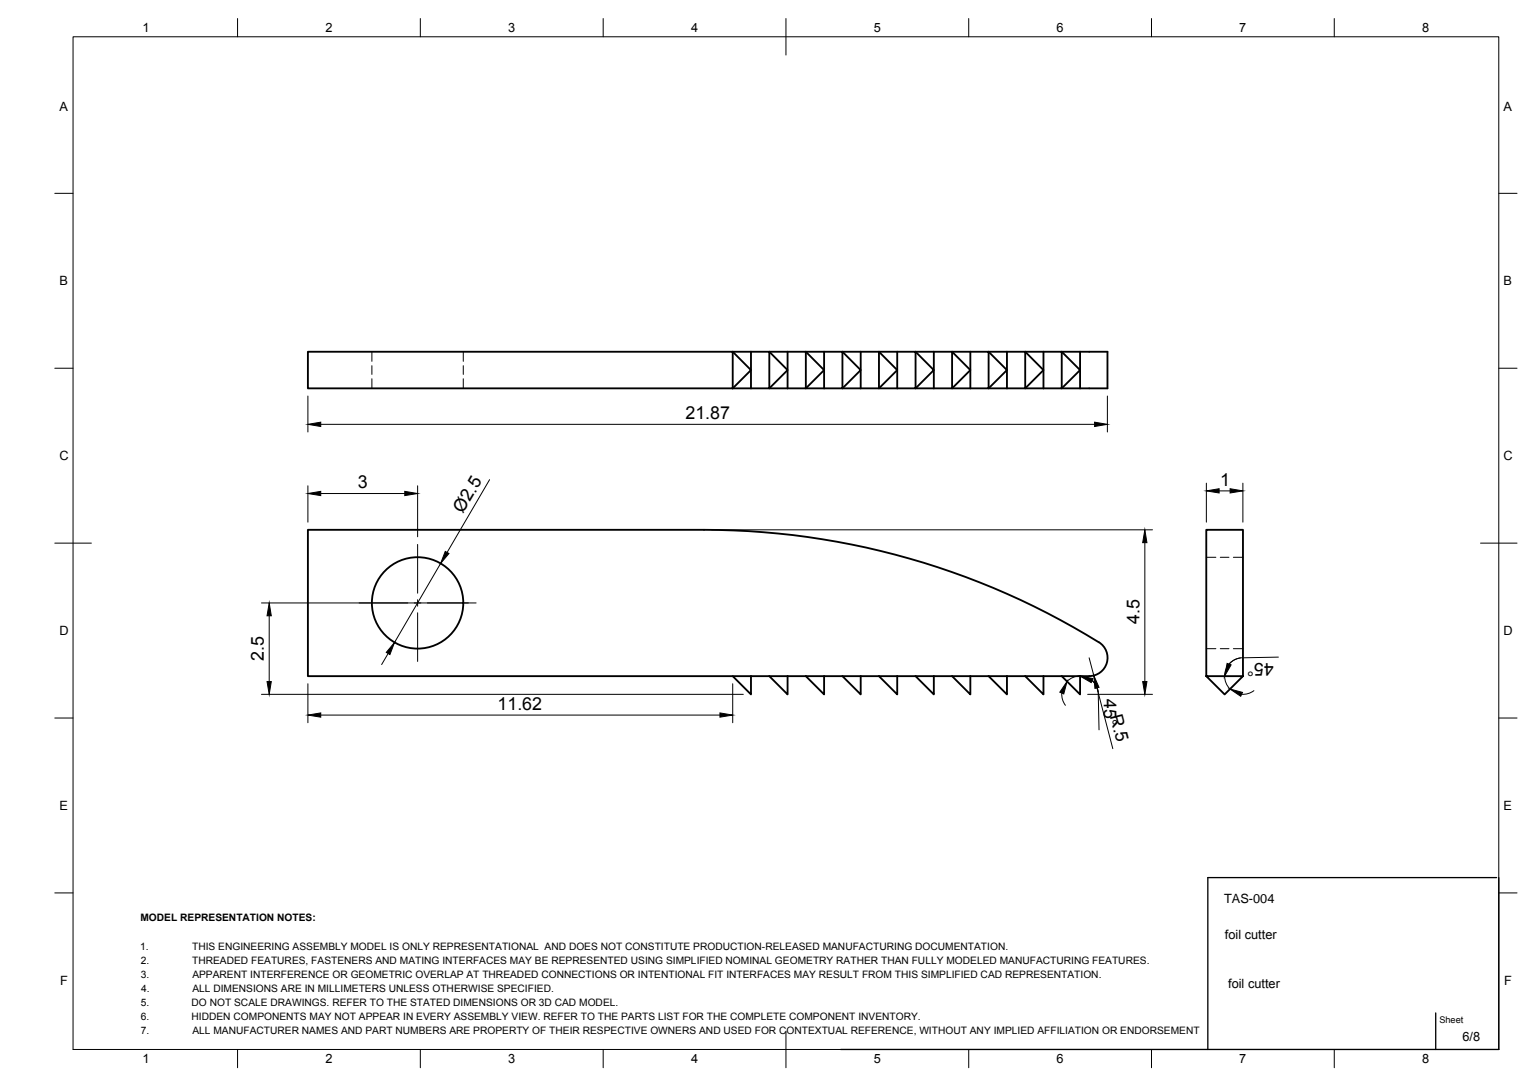
ISO-10303-21;
HEADER;
/* Generated by software containing ST-Developer
 * from STEP Tools, Inc. (www.steptools.com) 
 */

FILE_DESCRIPTION(
/* description */ ('STEP AP214'),
/* implementation_level */ '2;1');

FILE_NAME(
/* name */ 'foil cutter.step',
/* time_stamp */ '2026-11-04T19:48:07-08:00',
/* author */ (''),
/* organization */ (''),
/* preprocessor_version */ 'ST-DEVELOPER v20.2',
/* originating_system */ 'Autodesk Translation Framework v15.17.0.0',
/* authorisation */ '');

FILE_SCHEMA (('AUTOMOTIVE_DESIGN { 1 0 10303 214 3 1 1 }'));
ENDSEC;

DATA;
#10=MECHANICAL_DESIGN_GEOMETRIC_PRESENTATION_REPRESENTATION('',(#62),#9561);
#50=SHAPE_REPRESENTATION_RELATIONSHIP('SRR','None',#9590,#56);
#56=ADVANCED_BREP_SHAPE_REPRESENTATION('',(#68),#9558);
#62=STYLED_ITEM('',(#9626),#68);
#68=MANIFOLD_SOLID_BREP('Body1',#2408);
#84=FACE_BOUND('',#444,.T.);
#85=FACE_BOUND('',#446,.T.);
#135=PLANE('',#2617);
#136=PLANE('',#2618);
#137=PLANE('',#2619);
#138=PLANE('',#2620);
#139=PLANE('',#2621);
#140=PLANE('',#2622);
#141=PLANE('',#2623);
#142=PLANE('',#2624);
#143=PLANE('',#2625);
#144=PLANE('',#2626);
#145=PLANE('',#2627);
#146=PLANE('',#2628);
#147=PLANE('',#2629);
#148=PLANE('',#2630);
#149=PLANE('',#2633);
#150=PLANE('',#2638);
#151=PLANE('',#2639);
#152=PLANE('',#2640);
#153=PLANE('',#2641);
#154=PLANE('',#2642);
#155=PLANE('',#2643);
#156=PLANE('',#2644);
#157=PLANE('',#2645);
#158=PLANE('',#2646);
#159=PLANE('',#2647);
#160=PLANE('',#2648);
#161=PLANE('',#2649);
#162=PLANE('',#2650);
#163=PLANE('',#2651);
#164=PLANE('',#2652);
#165=PLANE('',#2653);
#166=PLANE('',#2654);
#167=PLANE('',#2655);
#168=PLANE('',#2656);
#169=PLANE('',#2657);
#170=PLANE('',#2658);
#171=PLANE('',#2659);
#172=PLANE('',#2660);
#173=PLANE('',#2661);
#174=PLANE('',#2662);
#175=PLANE('',#2663);
#176=PLANE('',#2664);
#177=PLANE('',#2665);
#178=PLANE('',#2666);
#179=PLANE('',#2667);
#180=PLANE('',#2668);
#181=PLANE('',#2669);
#182=PLANE('',#2670);
#183=PLANE('',#2671);
#184=PLANE('',#2672);
#185=PLANE('',#2673);
#186=PLANE('',#2674);
#187=PLANE('',#2675);
#188=PLANE('',#2676);
#189=PLANE('',#2677);
#273=FACE_OUTER_BOUND('',#429,.T.);
#274=FACE_OUTER_BOUND('',#430,.T.);
#275=FACE_OUTER_BOUND('',#431,.T.);
#276=FACE_OUTER_BOUND('',#432,.T.);
#277=FACE_OUTER_BOUND('',#433,.T.);
#278=FACE_OUTER_BOUND('',#434,.T.);
#279=FACE_OUTER_BOUND('',#435,.T.);
#280=FACE_OUTER_BOUND('',#436,.T.);
#281=FACE_OUTER_BOUND('',#437,.T.);
#282=FACE_OUTER_BOUND('',#438,.T.);
#283=FACE_OUTER_BOUND('',#439,.T.);
#284=FACE_OUTER_BOUND('',#440,.T.);
#285=FACE_OUTER_BOUND('',#441,.T.);
#286=FACE_OUTER_BOUND('',#442,.T.);
#287=FACE_OUTER_BOUND('',#443,.T.);
#288=FACE_OUTER_BOUND('',#445,.T.);
#289=FACE_OUTER_BOUND('',#447,.T.);
#290=FACE_OUTER_BOUND('',#448,.T.);
#291=FACE_OUTER_BOUND('',#449,.T.);
#292=FACE_OUTER_BOUND('',#450,.T.);
#293=FACE_OUTER_BOUND('',#451,.T.);
#294=FACE_OUTER_BOUND('',#452,.T.);
#295=FACE_OUTER_BOUND('',#453,.T.);
#296=FACE_OUTER_BOUND('',#454,.T.);
#297=FACE_OUTER_BOUND('',#455,.T.);
#298=FACE_OUTER_BOUND('',#456,.T.);
#299=FACE_OUTER_BOUND('',#457,.T.);
#300=FACE_OUTER_BOUND('',#458,.T.);
#301=FACE_OUTER_BOUND('',#459,.T.);
#302=FACE_OUTER_BOUND('',#460,.T.);
#303=FACE_OUTER_BOUND('',#461,.T.);
#304=FACE_OUTER_BOUND('',#462,.T.);
#305=FACE_OUTER_BOUND('',#463,.T.);
#306=FACE_OUTER_BOUND('',#464,.T.);
#307=FACE_OUTER_BOUND('',#465,.T.);
#308=FACE_OUTER_BOUND('',#466,.T.);
#309=FACE_OUTER_BOUND('',#467,.T.);
#310=FACE_OUTER_BOUND('',#468,.T.);
#311=FACE_OUTER_BOUND('',#469,.T.);
#312=FACE_OUTER_BOUND('',#470,.T.);
#313=FACE_OUTER_BOUND('',#471,.T.);
#314=FACE_OUTER_BOUND('',#472,.T.);
#315=FACE_OUTER_BOUND('',#473,.T.);
#316=FACE_OUTER_BOUND('',#474,.T.);
#317=FACE_OUTER_BOUND('',#475,.T.);
#318=FACE_OUTER_BOUND('',#476,.T.);
#319=FACE_OUTER_BOUND('',#477,.T.);
#320=FACE_OUTER_BOUND('',#478,.T.);
#321=FACE_OUTER_BOUND('',#479,.T.);
#322=FACE_OUTER_BOUND('',#480,.T.);
#323=FACE_OUTER_BOUND('',#481,.T.);
#324=FACE_OUTER_BOUND('',#482,.T.);
#325=FACE_OUTER_BOUND('',#483,.T.);
#326=FACE_OUTER_BOUND('',#484,.T.);
#327=FACE_OUTER_BOUND('',#485,.T.);
#328=FACE_OUTER_BOUND('',#486,.T.);
#329=FACE_OUTER_BOUND('',#487,.T.);
#330=FACE_OUTER_BOUND('',#488,.T.);
#429=EDGE_LOOP('',(#1983,#1984,#1985,#1986));
#430=EDGE_LOOP('',(#1987,#1988,#1989,#1990));
#431=EDGE_LOOP('',(#1991,#1992,#1993,#1994));
#432=EDGE_LOOP('',(#1995,#1996,#1997,#1998));
#433=EDGE_LOOP('',(#1999,#2000,#2001,#2002));
#434=EDGE_LOOP('',(#2003,#2004,#2005,#2006));
#435=EDGE_LOOP('',(#2007,#2008,#2009,#2010));
#436=EDGE_LOOP('',(#2011,#2012,#2013,#2014));
#437=EDGE_LOOP('',(#2015,#2016,#2017,#2018));
#438=EDGE_LOOP('',(#2019,#2020,#2021,#2022));
#439=EDGE_LOOP('',(#2023,#2024,#2025,#2026));
#440=EDGE_LOOP('',(#2027,#2028,#2029,#2030));
#441=EDGE_LOOP('',(#2031,#2032,#2033,#2034));
#442=EDGE_LOOP('',(#2035,#2036,#2037,#2038));
#443=EDGE_LOOP('',(#2039,#2040,#2041,#2042,#2043,#2044,#2045,#2046,#2047,
#2048,#2049,#2050,#2051,#2052,#2053,#2054,#2055,#2056,#2057,#2058,#2059,
#2060,#2061,#2062,#2063));
#444=EDGE_LOOP('',(#2064));
#445=EDGE_LOOP('',(#2065,#2066,#2067,#2068,#2069,#2070,#2071,#2072,#2073,
#2074,#2075,#2076,#2077,#2078,#2079,#2080,#2081,#2082,#2083,#2084,#2085,
#2086,#2087,#2088,#2089));
#446=EDGE_LOOP('',(#2090));
#447=EDGE_LOOP('',(#2091,#2092,#2093,#2094));
#448=EDGE_LOOP('',(#2095,#2096,#2097,#2098));
#449=EDGE_LOOP('',(#2099,#2100,#2101));
#450=EDGE_LOOP('',(#2102,#2103,#2104));
#451=EDGE_LOOP('',(#2105,#2106,#2107));
#452=EDGE_LOOP('',(#2108,#2109,#2110));
#453=EDGE_LOOP('',(#2111,#2112,#2113));
#454=EDGE_LOOP('',(#2114,#2115,#2116));
#455=EDGE_LOOP('',(#2117,#2118,#2119));
#456=EDGE_LOOP('',(#2120,#2121,#2122));
#457=EDGE_LOOP('',(#2123,#2124,#2125));
#458=EDGE_LOOP('',(#2126,#2127,#2128));
#459=EDGE_LOOP('',(#2129,#2130,#2131));
#460=EDGE_LOOP('',(#2132,#2133,#2134));
#461=EDGE_LOOP('',(#2135,#2136,#2137));
#462=EDGE_LOOP('',(#2138,#2139,#2140));
#463=EDGE_LOOP('',(#2141,#2142,#2143));
#464=EDGE_LOOP('',(#2144,#2145,#2146));
#465=EDGE_LOOP('',(#2147,#2148,#2149));
#466=EDGE_LOOP('',(#2150,#2151,#2152));
#467=EDGE_LOOP('',(#2153,#2154,#2155));
#468=EDGE_LOOP('',(#2156,#2157,#2158));
#469=EDGE_LOOP('',(#2159,#2160,#2161));
#470=EDGE_LOOP('',(#2162,#2163,#2164));
#471=EDGE_LOOP('',(#2165,#2166,#2167));
#472=EDGE_LOOP('',(#2168,#2169,#2170));
#473=EDGE_LOOP('',(#2171,#2172,#2173));
#474=EDGE_LOOP('',(#2174,#2175,#2176));
#475=EDGE_LOOP('',(#2177,#2178,#2179));
#476=EDGE_LOOP('',(#2180,#2181,#2182));
#477=EDGE_LOOP('',(#2183,#2184,#2185));
#478=EDGE_LOOP('',(#2186,#2187,#2188));
#479=EDGE_LOOP('',(#2189,#2190,#2191));
#480=EDGE_LOOP('',(#2192,#2193,#2194));
#481=EDGE_LOOP('',(#2195,#2196,#2197));
#482=EDGE_LOOP('',(#2198,#2199,#2200));
#483=EDGE_LOOP('',(#2201,#2202,#2203));
#484=EDGE_LOOP('',(#2204,#2205,#2206));
#485=EDGE_LOOP('',(#2207,#2208,#2209));
#486=EDGE_LOOP('',(#2210,#2211,#2212));
#487=EDGE_LOOP('',(#2213,#2214,#2215));
#488=EDGE_LOOP('',(#2216,#2217,#2218));
#631=LINE('',#9288,#881);
#632=LINE('',#9293,#882);
#633=LINE('',#9295,#883);
#634=LINE('',#9297,#884);
#635=LINE('',#9298,#885);
#636=LINE('',#9302,#886);
#637=LINE('',#9304,#887);
#638=LINE('',#9306,#888);
#639=LINE('',#9307,#889);
#640=LINE('',#9311,#890);
#641=LINE('',#9313,#891);
#642=LINE('',#9315,#892);
#643=LINE('',#9316,#893);
#644=LINE('',#9320,#894);
#645=LINE('',#9322,#895);
#646=LINE('',#9324,#896);
#647=LINE('',#9325,#897);
#648=LINE('',#9329,#898);
#649=LINE('',#9331,#899);
#650=LINE('',#9333,#900);
#651=LINE('',#9334,#901);
#652=LINE('',#9338,#902);
#653=LINE('',#9340,#903);
#654=LINE('',#9342,#904);
#655=LINE('',#9343,#905);
#656=LINE('',#9347,#906);
#657=LINE('',#9349,#907);
#658=LINE('',#9351,#908);
#659=LINE('',#9352,#909);
#660=LINE('',#9356,#910);
#661=LINE('',#9358,#911);
#662=LINE('',#9360,#912);
#663=LINE('',#9361,#913);
#664=LINE('',#9365,#914);
#665=LINE('',#9367,#915);
#666=LINE('',#9369,#916);
#667=LINE('',#9370,#917);
#668=LINE('',#9374,#918);
#669=LINE('',#9376,#919);
#670=LINE('',#9378,#920);
#671=LINE('',#9379,#921);
#672=LINE('',#9383,#922);
#673=LINE('',#9385,#923);
#674=LINE('',#9387,#924);
#675=LINE('',#9388,#925);
#676=LINE('',#9391,#926);
#677=LINE('',#9393,#927);
#678=LINE('',#9394,#928);
#679=LINE('',#9397,#929);
#680=LINE('',#9399,#930);
#681=LINE('',#9400,#931);
#682=LINE('',#9402,#932);
#683=LINE('',#9403,#933);
#684=LINE('',#9404,#934);
#685=LINE('',#9405,#935);
#686=LINE('',#9406,#936);
#687=LINE('',#9407,#937);
#688=LINE('',#9408,#938);
#689=LINE('',#9409,#939);
#690=LINE('',#9410,#940);
#691=LINE('',#9411,#941);
#692=LINE('',#9416,#942);
#693=LINE('',#9417,#943);
#694=LINE('',#9418,#944);
#695=LINE('',#9419,#945);
#696=LINE('',#9420,#946);
#697=LINE('',#9421,#947);
#698=LINE('',#9422,#948);
#699=LINE('',#9423,#949);
#700=LINE('',#9424,#950);
#701=LINE('',#9425,#951);
#702=LINE('',#9430,#952);
#703=LINE('',#9434,#953);
#704=LINE('',#9435,#954);
#705=LINE('',#9437,#955);
#706=LINE('',#9439,#956);
#707=LINE('',#9443,#957);
#708=LINE('',#9444,#958);
#709=LINE('',#9446,#959);
#710=LINE('',#9448,#960);
#711=LINE('',#9452,#961);
#712=LINE('',#9453,#962);
#713=LINE('',#9455,#963);
#714=LINE('',#9457,#964);
#715=LINE('',#9461,#965);
#716=LINE('',#9462,#966);
#717=LINE('',#9464,#967);
#718=LINE('',#9466,#968);
#719=LINE('',#9470,#969);
#720=LINE('',#9471,#970);
#721=LINE('',#9473,#971);
#722=LINE('',#9475,#972);
#723=LINE('',#9479,#973);
#724=LINE('',#9480,#974);
#725=LINE('',#9482,#975);
#726=LINE('',#9484,#976);
#727=LINE('',#9488,#977);
#728=LINE('',#9489,#978);
#729=LINE('',#9491,#979);
#730=LINE('',#9493,#980);
#731=LINE('',#9497,#981);
#732=LINE('',#9498,#982);
#733=LINE('',#9500,#983);
#734=LINE('',#9502,#984);
#735=LINE('',#9506,#985);
#736=LINE('',#9507,#986);
#737=LINE('',#9509,#987);
#738=LINE('',#9511,#988);
#739=LINE('',#9515,#989);
#740=LINE('',#9516,#990);
#741=LINE('',#9518,#991);
#742=LINE('',#9520,#992);
#881=VECTOR('',#3108,1.25);
#882=VECTOR('',#3113,1000.);
#883=VECTOR('',#3114,1000.);
#884=VECTOR('',#3115,1000.);
#885=VECTOR('',#3116,1000.);
#886=VECTOR('',#3119,1000.);
#887=VECTOR('',#3120,1000.);
#888=VECTOR('',#3121,1000.);
#889=VECTOR('',#3122,1000.);
#890=VECTOR('',#3125,1000.);
#891=VECTOR('',#3126,1000.);
#892=VECTOR('',#3127,1000.);
#893=VECTOR('',#3128,1000.);
#894=VECTOR('',#3131,1000.);
#895=VECTOR('',#3132,1000.);
#896=VECTOR('',#3133,1000.);
#897=VECTOR('',#3134,1000.);
#898=VECTOR('',#3137,1000.);
#899=VECTOR('',#3138,1000.);
#900=VECTOR('',#3139,1000.);
#901=VECTOR('',#3140,1000.);
#902=VECTOR('',#3143,1000.);
#903=VECTOR('',#3144,1000.);
#904=VECTOR('',#3145,1000.);
#905=VECTOR('',#3146,1000.);
#906=VECTOR('',#3149,1000.);
#907=VECTOR('',#3150,1000.);
#908=VECTOR('',#3151,1000.);
#909=VECTOR('',#3152,1000.);
#910=VECTOR('',#3155,1000.);
#911=VECTOR('',#3156,1000.);
#912=VECTOR('',#3157,1000.);
#913=VECTOR('',#3158,1000.);
#914=VECTOR('',#3161,1000.);
#915=VECTOR('',#3162,1000.);
#916=VECTOR('',#3163,1000.);
#917=VECTOR('',#3164,1000.);
#918=VECTOR('',#3167,1000.);
#919=VECTOR('',#3168,1000.);
#920=VECTOR('',#3169,1000.);
#921=VECTOR('',#3170,1000.);
#922=VECTOR('',#3173,1000.);
#923=VECTOR('',#3174,1000.);
#924=VECTOR('',#3175,1000.);
#925=VECTOR('',#3176,1000.);
#926=VECTOR('',#3179,1000.);
#927=VECTOR('',#3180,1000.);
#928=VECTOR('',#3181,1000.);
#929=VECTOR('',#3184,1000.);
#930=VECTOR('',#3185,1000.);
#931=VECTOR('',#3186,1000.);
#932=VECTOR('',#3189,1000.);
#933=VECTOR('',#3190,1000.);
#934=VECTOR('',#3191,1000.);
#935=VECTOR('',#3192,1000.);
#936=VECTOR('',#3193,1000.);
#937=VECTOR('',#3194,1000.);
#938=VECTOR('',#3195,1000.);
#939=VECTOR('',#3196,1000.);
#940=VECTOR('',#3197,1000.);
#941=VECTOR('',#3198,1000.);
#942=VECTOR('',#3205,1000.);
#943=VECTOR('',#3206,1000.);
#944=VECTOR('',#3207,1000.);
#945=VECTOR('',#3208,1000.);
#946=VECTOR('',#3209,1000.);
#947=VECTOR('',#3210,1000.);
#948=VECTOR('',#3211,1000.);
#949=VECTOR('',#3212,1000.);
#950=VECTOR('',#3213,1000.);
#951=VECTOR('',#3214,1000.);
#952=VECTOR('',#3221,1000.);
#953=VECTOR('',#3226,1000.);
#954=VECTOR('',#3227,1000.);
#955=VECTOR('',#3230,1000.);
#956=VECTOR('',#3233,1000.);
#957=VECTOR('',#3238,1000.);
#958=VECTOR('',#3239,1000.);
#959=VECTOR('',#3242,1000.);
#960=VECTOR('',#3245,1000.);
#961=VECTOR('',#3250,1000.);
#962=VECTOR('',#3251,1000.);
#963=VECTOR('',#3254,1000.);
#964=VECTOR('',#3257,1000.);
#965=VECTOR('',#3262,1000.);
#966=VECTOR('',#3263,1000.);
#967=VECTOR('',#3266,1000.);
#968=VECTOR('',#3269,1000.);
#969=VECTOR('',#3274,1000.);
#970=VECTOR('',#3275,1000.);
#971=VECTOR('',#3278,1000.);
#972=VECTOR('',#3281,1000.);
#973=VECTOR('',#3286,1000.);
#974=VECTOR('',#3287,1000.);
#975=VECTOR('',#3290,1000.);
#976=VECTOR('',#3293,1000.);
#977=VECTOR('',#3298,1000.);
#978=VECTOR('',#3299,1000.);
#979=VECTOR('',#3302,1000.);
#980=VECTOR('',#3305,1000.);
#981=VECTOR('',#3310,1000.);
#982=VECTOR('',#3311,1000.);
#983=VECTOR('',#3314,1000.);
#984=VECTOR('',#3317,1000.);
#985=VECTOR('',#3322,1000.);
#986=VECTOR('',#3323,1000.);
#987=VECTOR('',#3326,1000.);
#988=VECTOR('',#3329,1000.);
#989=VECTOR('',#3334,1000.);
#990=VECTOR('',#3335,1000.);
#991=VECTOR('',#3338,1000.);
#992=VECTOR('',#3341,1000.);
#1051=CIRCLE('',#2615,1.25);
#1052=CIRCLE('',#2616,1.25);
#1053=CIRCLE('',#2631,20.5);
#1054=CIRCLE('',#2632,0.5);
#1055=CIRCLE('',#2634,0.5);
#1056=CIRCLE('',#2635,20.5);
#1193=VERTEX_POINT('',#9285);
#1194=VERTEX_POINT('',#9287);
#1195=VERTEX_POINT('',#9291);
#1196=VERTEX_POINT('',#9292);
#1197=VERTEX_POINT('',#9294);
#1198=VERTEX_POINT('',#9296);
#1199=VERTEX_POINT('',#9300);
#1200=VERTEX_POINT('',#9301);
#1201=VERTEX_POINT('',#9303);
#1202=VERTEX_POINT('',#9305);
#1203=VERTEX_POINT('',#9309);
#1204=VERTEX_POINT('',#9310);
#1205=VERTEX_POINT('',#9312);
#1206=VERTEX_POINT('',#9314);
#1207=VERTEX_POINT('',#9318);
#1208=VERTEX_POINT('',#9319);
#1209=VERTEX_POINT('',#9321);
#1210=VERTEX_POINT('',#9323);
#1211=VERTEX_POINT('',#9327);
#1212=VERTEX_POINT('',#9328);
#1213=VERTEX_POINT('',#9330);
#1214=VERTEX_POINT('',#9332);
#1215=VERTEX_POINT('',#9336);
#1216=VERTEX_POINT('',#9337);
#1217=VERTEX_POINT('',#9339);
#1218=VERTEX_POINT('',#9341);
#1219=VERTEX_POINT('',#9345);
#1220=VERTEX_POINT('',#9346);
#1221=VERTEX_POINT('',#9348);
#1222=VERTEX_POINT('',#9350);
#1223=VERTEX_POINT('',#9354);
#1224=VERTEX_POINT('',#9355);
#1225=VERTEX_POINT('',#9357);
#1226=VERTEX_POINT('',#9359);
#1227=VERTEX_POINT('',#9363);
#1228=VERTEX_POINT('',#9364);
#1229=VERTEX_POINT('',#9366);
#1230=VERTEX_POINT('',#9368);
#1231=VERTEX_POINT('',#9372);
#1232=VERTEX_POINT('',#9373);
#1233=VERTEX_POINT('',#9375);
#1234=VERTEX_POINT('',#9377);
#1235=VERTEX_POINT('',#9381);
#1236=VERTEX_POINT('',#9382);
#1237=VERTEX_POINT('',#9384);
#1238=VERTEX_POINT('',#9386);
#1239=VERTEX_POINT('',#9390);
#1240=VERTEX_POINT('',#9392);
#1241=VERTEX_POINT('',#9396);
#1242=VERTEX_POINT('',#9398);
#1243=VERTEX_POINT('',#9412);
#1244=VERTEX_POINT('',#9426);
#1245=VERTEX_POINT('',#9433);
#1246=VERTEX_POINT('',#9442);
#1247=VERTEX_POINT('',#9451);
#1248=VERTEX_POINT('',#9460);
#1249=VERTEX_POINT('',#9469);
#1250=VERTEX_POINT('',#9478);
#1251=VERTEX_POINT('',#9487);
#1252=VERTEX_POINT('',#9496);
#1253=VERTEX_POINT('',#9505);
#1254=VERTEX_POINT('',#9514);
#1459=EDGE_CURVE('',#1193,#1193,#1051,.T.);
#1460=EDGE_CURVE('',#1193,#1194,#631,.T.);
#1461=EDGE_CURVE('',#1194,#1194,#1052,.T.);
#1462=EDGE_CURVE('',#1195,#1196,#632,.T.);
#1463=EDGE_CURVE('',#1196,#1197,#633,.T.);
#1464=EDGE_CURVE('',#1198,#1197,#634,.T.);
#1465=EDGE_CURVE('',#1195,#1198,#635,.T.);
#1466=EDGE_CURVE('',#1199,#1200,#636,.T.);
#1467=EDGE_CURVE('',#1201,#1199,#637,.T.);
#1468=EDGE_CURVE('',#1201,#1202,#638,.T.);
#1469=EDGE_CURVE('',#1202,#1200,#639,.T.);
#1470=EDGE_CURVE('',#1203,#1204,#640,.T.);
#1471=EDGE_CURVE('',#1205,#1203,#641,.T.);
#1472=EDGE_CURVE('',#1205,#1206,#642,.T.);
#1473=EDGE_CURVE('',#1206,#1204,#643,.T.);
#1474=EDGE_CURVE('',#1207,#1208,#644,.T.);
#1475=EDGE_CURVE('',#1209,#1207,#645,.T.);
#1476=EDGE_CURVE('',#1209,#1210,#646,.T.);
#1477=EDGE_CURVE('',#1210,#1208,#647,.T.);
#1478=EDGE_CURVE('',#1211,#1212,#648,.T.);
#1479=EDGE_CURVE('',#1213,#1211,#649,.T.);
#1480=EDGE_CURVE('',#1213,#1214,#650,.T.);
#1481=EDGE_CURVE('',#1214,#1212,#651,.T.);
#1482=EDGE_CURVE('',#1215,#1216,#652,.T.);
#1483=EDGE_CURVE('',#1217,#1215,#653,.T.);
#1484=EDGE_CURVE('',#1217,#1218,#654,.T.);
#1485=EDGE_CURVE('',#1218,#1216,#655,.T.);
#1486=EDGE_CURVE('',#1219,#1220,#656,.T.);
#1487=EDGE_CURVE('',#1221,#1219,#657,.T.);
#1488=EDGE_CURVE('',#1221,#1222,#658,.T.);
#1489=EDGE_CURVE('',#1222,#1220,#659,.T.);
#1490=EDGE_CURVE('',#1223,#1224,#660,.T.);
#1491=EDGE_CURVE('',#1225,#1223,#661,.T.);
#1492=EDGE_CURVE('',#1225,#1226,#662,.T.);
#1493=EDGE_CURVE('',#1226,#1224,#663,.T.);
#1494=EDGE_CURVE('',#1227,#1228,#664,.T.);
#1495=EDGE_CURVE('',#1229,#1227,#665,.T.);
#1496=EDGE_CURVE('',#1229,#1230,#666,.T.);
#1497=EDGE_CURVE('',#1230,#1228,#667,.T.);
#1498=EDGE_CURVE('',#1231,#1232,#668,.T.);
#1499=EDGE_CURVE('',#1231,#1233,#669,.T.);
#1500=EDGE_CURVE('',#1233,#1234,#670,.T.);
#1501=EDGE_CURVE('',#1234,#1232,#671,.T.);
#1502=EDGE_CURVE('',#1235,#1236,#672,.T.);
#1503=EDGE_CURVE('',#1237,#1235,#673,.T.);
#1504=EDGE_CURVE('',#1238,#1237,#674,.T.);
#1505=EDGE_CURVE('',#1238,#1236,#675,.T.);
#1506=EDGE_CURVE('',#1239,#1237,#676,.T.);
#1507=EDGE_CURVE('',#1240,#1239,#677,.T.);
#1508=EDGE_CURVE('',#1240,#1238,#678,.T.);
#1509=EDGE_CURVE('',#1239,#1241,#679,.T.);
#1510=EDGE_CURVE('',#1241,#1242,#680,.T.);
#1511=EDGE_CURVE('',#1240,#1242,#681,.T.);
#1512=EDGE_CURVE('',#1233,#1197,#682,.T.);
#1513=EDGE_CURVE('',#1196,#1200,#683,.T.);
#1514=EDGE_CURVE('',#1202,#1204,#684,.T.);
#1515=EDGE_CURVE('',#1206,#1208,#685,.T.);
#1516=EDGE_CURVE('',#1210,#1212,#686,.T.);
#1517=EDGE_CURVE('',#1214,#1216,#687,.T.);
#1518=EDGE_CURVE('',#1218,#1220,#688,.T.);
#1519=EDGE_CURVE('',#1222,#1224,#689,.T.);
#1520=EDGE_CURVE('',#1226,#1228,#690,.T.);
#1521=EDGE_CURVE('',#1230,#1236,#691,.T.);
#1522=EDGE_CURVE('',#1242,#1243,#1053,.T.);
#1523=EDGE_CURVE('',#1243,#1234,#1054,.T.);
#1524=EDGE_CURVE('',#1235,#1229,#692,.T.);
#1525=EDGE_CURVE('',#1227,#1225,#693,.T.);
#1526=EDGE_CURVE('',#1223,#1221,#694,.T.);
#1527=EDGE_CURVE('',#1219,#1217,#695,.T.);
#1528=EDGE_CURVE('',#1215,#1213,#696,.T.);
#1529=EDGE_CURVE('',#1211,#1209,#697,.T.);
#1530=EDGE_CURVE('',#1207,#1205,#698,.T.);
#1531=EDGE_CURVE('',#1203,#1201,#699,.T.);
#1532=EDGE_CURVE('',#1199,#1195,#700,.T.);
#1533=EDGE_CURVE('',#1198,#1231,#701,.T.);
#1534=EDGE_CURVE('',#1232,#1244,#1055,.T.);
#1535=EDGE_CURVE('',#1244,#1241,#1056,.T.);
#1536=EDGE_CURVE('',#1244,#1243,#702,.T.);
#1537=EDGE_CURVE('',#1231,#1245,#703,.T.);
#1538=EDGE_CURVE('',#1245,#1233,#704,.T.);
#1539=EDGE_CURVE('',#1197,#1245,#705,.T.);
#1540=EDGE_CURVE('',#1198,#1245,#706,.T.);
#1541=EDGE_CURVE('',#1229,#1246,#707,.T.);
#1542=EDGE_CURVE('',#1246,#1230,#708,.T.);
#1543=EDGE_CURVE('',#1236,#1246,#709,.T.);
#1544=EDGE_CURVE('',#1235,#1246,#710,.T.);
#1545=EDGE_CURVE('',#1225,#1247,#711,.T.);
#1546=EDGE_CURVE('',#1247,#1226,#712,.T.);
#1547=EDGE_CURVE('',#1228,#1247,#713,.T.);
#1548=EDGE_CURVE('',#1227,#1247,#714,.T.);
#1549=EDGE_CURVE('',#1221,#1248,#715,.T.);
#1550=EDGE_CURVE('',#1248,#1222,#716,.T.);
#1551=EDGE_CURVE('',#1224,#1248,#717,.T.);
#1552=EDGE_CURVE('',#1223,#1248,#718,.T.);
#1553=EDGE_CURVE('',#1217,#1249,#719,.T.);
#1554=EDGE_CURVE('',#1249,#1218,#720,.T.);
#1555=EDGE_CURVE('',#1220,#1249,#721,.T.);
#1556=EDGE_CURVE('',#1219,#1249,#722,.T.);
#1557=EDGE_CURVE('',#1213,#1250,#723,.T.);
#1558=EDGE_CURVE('',#1250,#1214,#724,.T.);
#1559=EDGE_CURVE('',#1216,#1250,#725,.T.);
#1560=EDGE_CURVE('',#1215,#1250,#726,.T.);
#1561=EDGE_CURVE('',#1209,#1251,#727,.T.);
#1562=EDGE_CURVE('',#1251,#1210,#728,.T.);
#1563=EDGE_CURVE('',#1212,#1251,#729,.T.);
#1564=EDGE_CURVE('',#1211,#1251,#730,.T.);
#1565=EDGE_CURVE('',#1205,#1252,#731,.T.);
#1566=EDGE_CURVE('',#1252,#1206,#732,.T.);
#1567=EDGE_CURVE('',#1208,#1252,#733,.T.);
#1568=EDGE_CURVE('',#1207,#1252,#734,.T.);
#1569=EDGE_CURVE('',#1201,#1253,#735,.T.);
#1570=EDGE_CURVE('',#1253,#1202,#736,.T.);
#1571=EDGE_CURVE('',#1204,#1253,#737,.T.);
#1572=EDGE_CURVE('',#1203,#1253,#738,.T.);
#1573=EDGE_CURVE('',#1195,#1254,#739,.T.);
#1574=EDGE_CURVE('',#1254,#1196,#740,.T.);
#1575=EDGE_CURVE('',#1200,#1254,#741,.T.);
#1576=EDGE_CURVE('',#1199,#1254,#742,.T.);
#1983=ORIENTED_EDGE('',*,*,#1459,.T.);
#1984=ORIENTED_EDGE('',*,*,#1460,.T.);
#1985=ORIENTED_EDGE('',*,*,#1461,.F.);
#1986=ORIENTED_EDGE('',*,*,#1460,.F.);
#1987=ORIENTED_EDGE('',*,*,#1462,.T.);
#1988=ORIENTED_EDGE('',*,*,#1463,.T.);
#1989=ORIENTED_EDGE('',*,*,#1464,.F.);
#1990=ORIENTED_EDGE('',*,*,#1465,.F.);
#1991=ORIENTED_EDGE('',*,*,#1466,.F.);
#1992=ORIENTED_EDGE('',*,*,#1467,.F.);
#1993=ORIENTED_EDGE('',*,*,#1468,.T.);
#1994=ORIENTED_EDGE('',*,*,#1469,.T.);
#1995=ORIENTED_EDGE('',*,*,#1470,.F.);
#1996=ORIENTED_EDGE('',*,*,#1471,.F.);
#1997=ORIENTED_EDGE('',*,*,#1472,.T.);
#1998=ORIENTED_EDGE('',*,*,#1473,.T.);
#1999=ORIENTED_EDGE('',*,*,#1474,.F.);
#2000=ORIENTED_EDGE('',*,*,#1475,.F.);
#2001=ORIENTED_EDGE('',*,*,#1476,.T.);
#2002=ORIENTED_EDGE('',*,*,#1477,.T.);
#2003=ORIENTED_EDGE('',*,*,#1478,.F.);
#2004=ORIENTED_EDGE('',*,*,#1479,.F.);
#2005=ORIENTED_EDGE('',*,*,#1480,.T.);
#2006=ORIENTED_EDGE('',*,*,#1481,.T.);
#2007=ORIENTED_EDGE('',*,*,#1482,.F.);
#2008=ORIENTED_EDGE('',*,*,#1483,.F.);
#2009=ORIENTED_EDGE('',*,*,#1484,.T.);
#2010=ORIENTED_EDGE('',*,*,#1485,.T.);
#2011=ORIENTED_EDGE('',*,*,#1486,.F.);
#2012=ORIENTED_EDGE('',*,*,#1487,.F.);
#2013=ORIENTED_EDGE('',*,*,#1488,.T.);
#2014=ORIENTED_EDGE('',*,*,#1489,.T.);
#2015=ORIENTED_EDGE('',*,*,#1490,.F.);
#2016=ORIENTED_EDGE('',*,*,#1491,.F.);
#2017=ORIENTED_EDGE('',*,*,#1492,.T.);
#2018=ORIENTED_EDGE('',*,*,#1493,.T.);
#2019=ORIENTED_EDGE('',*,*,#1494,.F.);
#2020=ORIENTED_EDGE('',*,*,#1495,.F.);
#2021=ORIENTED_EDGE('',*,*,#1496,.T.);
#2022=ORIENTED_EDGE('',*,*,#1497,.T.);
#2023=ORIENTED_EDGE('',*,*,#1498,.F.);
#2024=ORIENTED_EDGE('',*,*,#1499,.T.);
#2025=ORIENTED_EDGE('',*,*,#1500,.T.);
#2026=ORIENTED_EDGE('',*,*,#1501,.T.);
#2027=ORIENTED_EDGE('',*,*,#1502,.F.);
#2028=ORIENTED_EDGE('',*,*,#1503,.F.);
#2029=ORIENTED_EDGE('',*,*,#1504,.F.);
#2030=ORIENTED_EDGE('',*,*,#1505,.T.);
#2031=ORIENTED_EDGE('',*,*,#1506,.F.);
#2032=ORIENTED_EDGE('',*,*,#1507,.F.);
#2033=ORIENTED_EDGE('',*,*,#1508,.T.);
#2034=ORIENTED_EDGE('',*,*,#1504,.T.);
#2035=ORIENTED_EDGE('',*,*,#1509,.T.);
#2036=ORIENTED_EDGE('',*,*,#1510,.T.);
#2037=ORIENTED_EDGE('',*,*,#1511,.F.);
#2038=ORIENTED_EDGE('',*,*,#1507,.T.);
#2039=ORIENTED_EDGE('',*,*,#1500,.F.);
#2040=ORIENTED_EDGE('',*,*,#1512,.T.);
#2041=ORIENTED_EDGE('',*,*,#1463,.F.);
#2042=ORIENTED_EDGE('',*,*,#1513,.T.);
#2043=ORIENTED_EDGE('',*,*,#1469,.F.);
#2044=ORIENTED_EDGE('',*,*,#1514,.T.);
#2045=ORIENTED_EDGE('',*,*,#1473,.F.);
#2046=ORIENTED_EDGE('',*,*,#1515,.T.);
#2047=ORIENTED_EDGE('',*,*,#1477,.F.);
#2048=ORIENTED_EDGE('',*,*,#1516,.T.);
#2049=ORIENTED_EDGE('',*,*,#1481,.F.);
#2050=ORIENTED_EDGE('',*,*,#1517,.T.);
#2051=ORIENTED_EDGE('',*,*,#1485,.F.);
#2052=ORIENTED_EDGE('',*,*,#1518,.T.);
#2053=ORIENTED_EDGE('',*,*,#1489,.F.);
#2054=ORIENTED_EDGE('',*,*,#1519,.T.);
#2055=ORIENTED_EDGE('',*,*,#1493,.F.);
#2056=ORIENTED_EDGE('',*,*,#1520,.T.);
#2057=ORIENTED_EDGE('',*,*,#1497,.F.);
#2058=ORIENTED_EDGE('',*,*,#1521,.T.);
#2059=ORIENTED_EDGE('',*,*,#1505,.F.);
#2060=ORIENTED_EDGE('',*,*,#1508,.F.);
#2061=ORIENTED_EDGE('',*,*,#1511,.T.);
#2062=ORIENTED_EDGE('',*,*,#1522,.T.);
#2063=ORIENTED_EDGE('',*,*,#1523,.T.);
#2064=ORIENTED_EDGE('',*,*,#1461,.T.);
#2065=ORIENTED_EDGE('',*,*,#1503,.T.);
#2066=ORIENTED_EDGE('',*,*,#1524,.T.);
#2067=ORIENTED_EDGE('',*,*,#1495,.T.);
#2068=ORIENTED_EDGE('',*,*,#1525,.T.);
#2069=ORIENTED_EDGE('',*,*,#1491,.T.);
#2070=ORIENTED_EDGE('',*,*,#1526,.T.);
#2071=ORIENTED_EDGE('',*,*,#1487,.T.);
#2072=ORIENTED_EDGE('',*,*,#1527,.T.);
#2073=ORIENTED_EDGE('',*,*,#1483,.T.);
#2074=ORIENTED_EDGE('',*,*,#1528,.T.);
#2075=ORIENTED_EDGE('',*,*,#1479,.T.);
#2076=ORIENTED_EDGE('',*,*,#1529,.T.);
#2077=ORIENTED_EDGE('',*,*,#1475,.T.);
#2078=ORIENTED_EDGE('',*,*,#1530,.T.);
#2079=ORIENTED_EDGE('',*,*,#1471,.T.);
#2080=ORIENTED_EDGE('',*,*,#1531,.T.);
#2081=ORIENTED_EDGE('',*,*,#1467,.T.);
#2082=ORIENTED_EDGE('',*,*,#1532,.T.);
#2083=ORIENTED_EDGE('',*,*,#1465,.T.);
#2084=ORIENTED_EDGE('',*,*,#1533,.T.);
#2085=ORIENTED_EDGE('',*,*,#1498,.T.);
#2086=ORIENTED_EDGE('',*,*,#1534,.T.);
#2087=ORIENTED_EDGE('',*,*,#1535,.T.);
#2088=ORIENTED_EDGE('',*,*,#1509,.F.);
#2089=ORIENTED_EDGE('',*,*,#1506,.T.);
#2090=ORIENTED_EDGE('',*,*,#1459,.F.);
#2091=ORIENTED_EDGE('',*,*,#1535,.F.);
#2092=ORIENTED_EDGE('',*,*,#1536,.T.);
#2093=ORIENTED_EDGE('',*,*,#1522,.F.);
#2094=ORIENTED_EDGE('',*,*,#1510,.F.);
#2095=ORIENTED_EDGE('',*,*,#1523,.F.);
#2096=ORIENTED_EDGE('',*,*,#1536,.F.);
#2097=ORIENTED_EDGE('',*,*,#1534,.F.);
#2098=ORIENTED_EDGE('',*,*,#1501,.F.);
#2099=ORIENTED_EDGE('',*,*,#1499,.F.);
#2100=ORIENTED_EDGE('',*,*,#1537,.T.);
#2101=ORIENTED_EDGE('',*,*,#1538,.T.);
#2102=ORIENTED_EDGE('',*,*,#1539,.F.);
#2103=ORIENTED_EDGE('',*,*,#1512,.F.);
#2104=ORIENTED_EDGE('',*,*,#1538,.F.);
#2105=ORIENTED_EDGE('',*,*,#1540,.F.);
#2106=ORIENTED_EDGE('',*,*,#1464,.T.);
#2107=ORIENTED_EDGE('',*,*,#1539,.T.);
#2108=ORIENTED_EDGE('',*,*,#1533,.F.);
#2109=ORIENTED_EDGE('',*,*,#1540,.T.);
#2110=ORIENTED_EDGE('',*,*,#1537,.F.);
#2111=ORIENTED_EDGE('',*,*,#1496,.F.);
#2112=ORIENTED_EDGE('',*,*,#1541,.T.);
#2113=ORIENTED_EDGE('',*,*,#1542,.T.);
#2114=ORIENTED_EDGE('',*,*,#1543,.F.);
#2115=ORIENTED_EDGE('',*,*,#1521,.F.);
#2116=ORIENTED_EDGE('',*,*,#1542,.F.);
#2117=ORIENTED_EDGE('',*,*,#1544,.F.);
#2118=ORIENTED_EDGE('',*,*,#1502,.T.);
#2119=ORIENTED_EDGE('',*,*,#1543,.T.);
#2120=ORIENTED_EDGE('',*,*,#1524,.F.);
#2121=ORIENTED_EDGE('',*,*,#1544,.T.);
#2122=ORIENTED_EDGE('',*,*,#1541,.F.);
#2123=ORIENTED_EDGE('',*,*,#1492,.F.);
#2124=ORIENTED_EDGE('',*,*,#1545,.T.);
#2125=ORIENTED_EDGE('',*,*,#1546,.T.);
#2126=ORIENTED_EDGE('',*,*,#1547,.F.);
#2127=ORIENTED_EDGE('',*,*,#1520,.F.);
#2128=ORIENTED_EDGE('',*,*,#1546,.F.);
#2129=ORIENTED_EDGE('',*,*,#1548,.F.);
#2130=ORIENTED_EDGE('',*,*,#1494,.T.);
#2131=ORIENTED_EDGE('',*,*,#1547,.T.);
#2132=ORIENTED_EDGE('',*,*,#1525,.F.);
#2133=ORIENTED_EDGE('',*,*,#1548,.T.);
#2134=ORIENTED_EDGE('',*,*,#1545,.F.);
#2135=ORIENTED_EDGE('',*,*,#1488,.F.);
#2136=ORIENTED_EDGE('',*,*,#1549,.T.);
#2137=ORIENTED_EDGE('',*,*,#1550,.T.);
#2138=ORIENTED_EDGE('',*,*,#1551,.F.);
#2139=ORIENTED_EDGE('',*,*,#1519,.F.);
#2140=ORIENTED_EDGE('',*,*,#1550,.F.);
#2141=ORIENTED_EDGE('',*,*,#1552,.F.);
#2142=ORIENTED_EDGE('',*,*,#1490,.T.);
#2143=ORIENTED_EDGE('',*,*,#1551,.T.);
#2144=ORIENTED_EDGE('',*,*,#1526,.F.);
#2145=ORIENTED_EDGE('',*,*,#1552,.T.);
#2146=ORIENTED_EDGE('',*,*,#1549,.F.);
#2147=ORIENTED_EDGE('',*,*,#1484,.F.);
#2148=ORIENTED_EDGE('',*,*,#1553,.T.);
#2149=ORIENTED_EDGE('',*,*,#1554,.T.);
#2150=ORIENTED_EDGE('',*,*,#1555,.F.);
#2151=ORIENTED_EDGE('',*,*,#1518,.F.);
#2152=ORIENTED_EDGE('',*,*,#1554,.F.);
#2153=ORIENTED_EDGE('',*,*,#1556,.F.);
#2154=ORIENTED_EDGE('',*,*,#1486,.T.);
#2155=ORIENTED_EDGE('',*,*,#1555,.T.);
#2156=ORIENTED_EDGE('',*,*,#1527,.F.);
#2157=ORIENTED_EDGE('',*,*,#1556,.T.);
#2158=ORIENTED_EDGE('',*,*,#1553,.F.);
#2159=ORIENTED_EDGE('',*,*,#1480,.F.);
#2160=ORIENTED_EDGE('',*,*,#1557,.T.);
#2161=ORIENTED_EDGE('',*,*,#1558,.T.);
#2162=ORIENTED_EDGE('',*,*,#1559,.F.);
#2163=ORIENTED_EDGE('',*,*,#1517,.F.);
#2164=ORIENTED_EDGE('',*,*,#1558,.F.);
#2165=ORIENTED_EDGE('',*,*,#1560,.F.);
#2166=ORIENTED_EDGE('',*,*,#1482,.T.);
#2167=ORIENTED_EDGE('',*,*,#1559,.T.);
#2168=ORIENTED_EDGE('',*,*,#1528,.F.);
#2169=ORIENTED_EDGE('',*,*,#1560,.T.);
#2170=ORIENTED_EDGE('',*,*,#1557,.F.);
#2171=ORIENTED_EDGE('',*,*,#1476,.F.);
#2172=ORIENTED_EDGE('',*,*,#1561,.T.);
#2173=ORIENTED_EDGE('',*,*,#1562,.T.);
#2174=ORIENTED_EDGE('',*,*,#1563,.F.);
#2175=ORIENTED_EDGE('',*,*,#1516,.F.);
#2176=ORIENTED_EDGE('',*,*,#1562,.F.);
#2177=ORIENTED_EDGE('',*,*,#1564,.F.);
#2178=ORIENTED_EDGE('',*,*,#1478,.T.);
#2179=ORIENTED_EDGE('',*,*,#1563,.T.);
#2180=ORIENTED_EDGE('',*,*,#1529,.F.);
#2181=ORIENTED_EDGE('',*,*,#1564,.T.);
#2182=ORIENTED_EDGE('',*,*,#1561,.F.);
#2183=ORIENTED_EDGE('',*,*,#1472,.F.);
#2184=ORIENTED_EDGE('',*,*,#1565,.T.);
#2185=ORIENTED_EDGE('',*,*,#1566,.T.);
#2186=ORIENTED_EDGE('',*,*,#1567,.F.);
#2187=ORIENTED_EDGE('',*,*,#1515,.F.);
#2188=ORIENTED_EDGE('',*,*,#1566,.F.);
#2189=ORIENTED_EDGE('',*,*,#1568,.F.);
#2190=ORIENTED_EDGE('',*,*,#1474,.T.);
#2191=ORIENTED_EDGE('',*,*,#1567,.T.);
#2192=ORIENTED_EDGE('',*,*,#1530,.F.);
#2193=ORIENTED_EDGE('',*,*,#1568,.T.);
#2194=ORIENTED_EDGE('',*,*,#1565,.F.);
#2195=ORIENTED_EDGE('',*,*,#1468,.F.);
#2196=ORIENTED_EDGE('',*,*,#1569,.T.);
#2197=ORIENTED_EDGE('',*,*,#1570,.T.);
#2198=ORIENTED_EDGE('',*,*,#1571,.F.);
#2199=ORIENTED_EDGE('',*,*,#1514,.F.);
#2200=ORIENTED_EDGE('',*,*,#1570,.F.);
#2201=ORIENTED_EDGE('',*,*,#1572,.F.);
#2202=ORIENTED_EDGE('',*,*,#1470,.T.);
#2203=ORIENTED_EDGE('',*,*,#1571,.T.);
#2204=ORIENTED_EDGE('',*,*,#1531,.F.);
#2205=ORIENTED_EDGE('',*,*,#1572,.T.);
#2206=ORIENTED_EDGE('',*,*,#1569,.F.);
#2207=ORIENTED_EDGE('',*,*,#1462,.F.);
#2208=ORIENTED_EDGE('',*,*,#1573,.T.);
#2209=ORIENTED_EDGE('',*,*,#1574,.T.);
#2210=ORIENTED_EDGE('',*,*,#1575,.F.);
#2211=ORIENTED_EDGE('',*,*,#1513,.F.);
#2212=ORIENTED_EDGE('',*,*,#1574,.F.);
#2213=ORIENTED_EDGE('',*,*,#1576,.F.);
#2214=ORIENTED_EDGE('',*,*,#1466,.T.);
#2215=ORIENTED_EDGE('',*,*,#1575,.T.);
#2216=ORIENTED_EDGE('',*,*,#1532,.F.);
#2217=ORIENTED_EDGE('',*,*,#1576,.T.);
#2218=ORIENTED_EDGE('',*,*,#1573,.F.);
#2257=CYLINDRICAL_SURFACE('',#2614,1.25);
#2258=CYLINDRICAL_SURFACE('',#2636,20.5);
#2259=CYLINDRICAL_SURFACE('',#2637,0.5);
#2341=ADVANCED_FACE('',(#273),#2257,.F.);
#2342=ADVANCED_FACE('',(#274),#135,.T.);
#2343=ADVANCED_FACE('',(#275),#136,.T.);
#2344=ADVANCED_FACE('',(#276),#137,.T.);
#2345=ADVANCED_FACE('',(#277),#138,.T.);
#2346=ADVANCED_FACE('',(#278),#139,.T.);
#2347=ADVANCED_FACE('',(#279),#140,.T.);
#2348=ADVANCED_FACE('',(#280),#141,.T.);
#2349=ADVANCED_FACE('',(#281),#142,.T.);
#2350=ADVANCED_FACE('',(#282),#143,.T.);
#2351=ADVANCED_FACE('',(#283),#144,.T.);
#2352=ADVANCED_FACE('',(#284),#145,.T.);
#2353=ADVANCED_FACE('',(#285),#146,.T.);
#2354=ADVANCED_FACE('',(#286),#147,.F.);
#2355=ADVANCED_FACE('',(#287,#84),#148,.F.);
#2356=ADVANCED_FACE('',(#288,#85),#149,.T.);
#2357=ADVANCED_FACE('',(#289),#2258,.T.);
#2358=ADVANCED_FACE('',(#290),#2259,.T.);
#2359=ADVANCED_FACE('',(#291),#150,.T.);
#2360=ADVANCED_FACE('',(#292),#151,.F.);
#2361=ADVANCED_FACE('',(#293),#152,.F.);
#2362=ADVANCED_FACE('',(#294),#153,.T.);
#2363=ADVANCED_FACE('',(#295),#154,.T.);
#2364=ADVANCED_FACE('',(#296),#155,.F.);
#2365=ADVANCED_FACE('',(#297),#156,.F.);
#2366=ADVANCED_FACE('',(#298),#157,.T.);
#2367=ADVANCED_FACE('',(#299),#158,.T.);
#2368=ADVANCED_FACE('',(#300),#159,.F.);
#2369=ADVANCED_FACE('',(#301),#160,.F.);
#2370=ADVANCED_FACE('',(#302),#161,.T.);
#2371=ADVANCED_FACE('',(#303),#162,.T.);
#2372=ADVANCED_FACE('',(#304),#163,.F.);
#2373=ADVANCED_FACE('',(#305),#164,.F.);
#2374=ADVANCED_FACE('',(#306),#165,.T.);
#2375=ADVANCED_FACE('',(#307),#166,.T.);
#2376=ADVANCED_FACE('',(#308),#167,.F.);
#2377=ADVANCED_FACE('',(#309),#168,.F.);
#2378=ADVANCED_FACE('',(#310),#169,.T.);
#2379=ADVANCED_FACE('',(#311),#170,.T.);
#2380=ADVANCED_FACE('',(#312),#171,.F.);
#2381=ADVANCED_FACE('',(#313),#172,.F.);
#2382=ADVANCED_FACE('',(#314),#173,.T.);
#2383=ADVANCED_FACE('',(#315),#174,.T.);
#2384=ADVANCED_FACE('',(#316),#175,.F.);
#2385=ADVANCED_FACE('',(#317),#176,.F.);
#2386=ADVANCED_FACE('',(#318),#177,.T.);
#2387=ADVANCED_FACE('',(#319),#178,.T.);
#2388=ADVANCED_FACE('',(#320),#179,.F.);
#2389=ADVANCED_FACE('',(#321),#180,.F.);
#2390=ADVANCED_FACE('',(#322),#181,.T.);
#2391=ADVANCED_FACE('',(#323),#182,.T.);
#2392=ADVANCED_FACE('',(#324),#183,.F.);
#2393=ADVANCED_FACE('',(#325),#184,.F.);
#2394=ADVANCED_FACE('',(#326),#185,.T.);
#2395=ADVANCED_FACE('',(#327),#186,.T.);
#2396=ADVANCED_FACE('',(#328),#187,.F.);
#2397=ADVANCED_FACE('',(#329),#188,.F.);
#2398=ADVANCED_FACE('',(#330),#189,.T.);
#2408=CLOSED_SHELL('',(#2341,#2342,#2343,#2344,#2345,#2346,#2347,#2348,
#2349,#2350,#2351,#2352,#2353,#2354,#2355,#2356,#2357,#2358,#2359,#2360,
#2361,#2362,#2363,#2364,#2365,#2366,#2367,#2368,#2369,#2370,#2371,#2372,
#2373,#2374,#2375,#2376,#2377,#2378,#2379,#2380,#2381,#2382,#2383,#2384,
#2385,#2386,#2387,#2388,#2389,#2390,#2391,#2392,#2393,#2394,#2395,#2396,
#2397,#2398));
#2613=AXIS2_PLACEMENT_3D('',#9283,#3102,#3103);
#2614=AXIS2_PLACEMENT_3D('',#9284,#3104,#3105);
#2615=AXIS2_PLACEMENT_3D('',#9286,#3106,#3107);
#2616=AXIS2_PLACEMENT_3D('',#9289,#3109,#3110);
#2617=AXIS2_PLACEMENT_3D('',#9290,#3111,#3112);
#2618=AXIS2_PLACEMENT_3D('',#9299,#3117,#3118);
#2619=AXIS2_PLACEMENT_3D('',#9308,#3123,#3124);
#2620=AXIS2_PLACEMENT_3D('',#9317,#3129,#3130);
#2621=AXIS2_PLACEMENT_3D('',#9326,#3135,#3136);
#2622=AXIS2_PLACEMENT_3D('',#9335,#3141,#3142);
#2623=AXIS2_PLACEMENT_3D('',#9344,#3147,#3148);
#2624=AXIS2_PLACEMENT_3D('',#9353,#3153,#3154);
#2625=AXIS2_PLACEMENT_3D('',#9362,#3159,#3160);
#2626=AXIS2_PLACEMENT_3D('',#9371,#3165,#3166);
#2627=AXIS2_PLACEMENT_3D('',#9380,#3171,#3172);
#2628=AXIS2_PLACEMENT_3D('',#9389,#3177,#3178);
#2629=AXIS2_PLACEMENT_3D('',#9395,#3182,#3183);
#2630=AXIS2_PLACEMENT_3D('',#9401,#3187,#3188);
#2631=AXIS2_PLACEMENT_3D('',#9413,#3199,#3200);
#2632=AXIS2_PLACEMENT_3D('',#9414,#3201,#3202);
#2633=AXIS2_PLACEMENT_3D('',#9415,#3203,#3204);
#2634=AXIS2_PLACEMENT_3D('',#9427,#3215,#3216);
#2635=AXIS2_PLACEMENT_3D('',#9428,#3217,#3218);
#2636=AXIS2_PLACEMENT_3D('',#9429,#3219,#3220);
#2637=AXIS2_PLACEMENT_3D('',#9431,#3222,#3223);
#2638=AXIS2_PLACEMENT_3D('',#9432,#3224,#3225);
#2639=AXIS2_PLACEMENT_3D('',#9436,#3228,#3229);
#2640=AXIS2_PLACEMENT_3D('',#9438,#3231,#3232);
#2641=AXIS2_PLACEMENT_3D('',#9440,#3234,#3235);
#2642=AXIS2_PLACEMENT_3D('',#9441,#3236,#3237);
#2643=AXIS2_PLACEMENT_3D('',#9445,#3240,#3241);
#2644=AXIS2_PLACEMENT_3D('',#9447,#3243,#3244);
#2645=AXIS2_PLACEMENT_3D('',#9449,#3246,#3247);
#2646=AXIS2_PLACEMENT_3D('',#9450,#3248,#3249);
#2647=AXIS2_PLACEMENT_3D('',#9454,#3252,#3253);
#2648=AXIS2_PLACEMENT_3D('',#9456,#3255,#3256);
#2649=AXIS2_PLACEMENT_3D('',#9458,#3258,#3259);
#2650=AXIS2_PLACEMENT_3D('',#9459,#3260,#3261);
#2651=AXIS2_PLACEMENT_3D('',#9463,#3264,#3265);
#2652=AXIS2_PLACEMENT_3D('',#9465,#3267,#3268);
#2653=AXIS2_PLACEMENT_3D('',#9467,#3270,#3271);
#2654=AXIS2_PLACEMENT_3D('',#9468,#3272,#3273);
#2655=AXIS2_PLACEMENT_3D('',#9472,#3276,#3277);
#2656=AXIS2_PLACEMENT_3D('',#9474,#3279,#3280);
#2657=AXIS2_PLACEMENT_3D('',#9476,#3282,#3283);
#2658=AXIS2_PLACEMENT_3D('',#9477,#3284,#3285);
#2659=AXIS2_PLACEMENT_3D('',#9481,#3288,#3289);
#2660=AXIS2_PLACEMENT_3D('',#9483,#3291,#3292);
#2661=AXIS2_PLACEMENT_3D('',#9485,#3294,#3295);
#2662=AXIS2_PLACEMENT_3D('',#9486,#3296,#3297);
#2663=AXIS2_PLACEMENT_3D('',#9490,#3300,#3301);
#2664=AXIS2_PLACEMENT_3D('',#9492,#3303,#3304);
#2665=AXIS2_PLACEMENT_3D('',#9494,#3306,#3307);
#2666=AXIS2_PLACEMENT_3D('',#9495,#3308,#3309);
#2667=AXIS2_PLACEMENT_3D('',#9499,#3312,#3313);
#2668=AXIS2_PLACEMENT_3D('',#9501,#3315,#3316);
#2669=AXIS2_PLACEMENT_3D('',#9503,#3318,#3319);
#2670=AXIS2_PLACEMENT_3D('',#9504,#3320,#3321);
#2671=AXIS2_PLACEMENT_3D('',#9508,#3324,#3325);
#2672=AXIS2_PLACEMENT_3D('',#9510,#3327,#3328);
#2673=AXIS2_PLACEMENT_3D('',#9512,#3330,#3331);
#2674=AXIS2_PLACEMENT_3D('',#9513,#3332,#3333);
#2675=AXIS2_PLACEMENT_3D('',#9517,#3336,#3337);
#2676=AXIS2_PLACEMENT_3D('',#9519,#3339,#3340);
#2677=AXIS2_PLACEMENT_3D('',#9521,#3342,#3343);
#3102=DIRECTION('axis',(0.,0.,1.));
#3103=DIRECTION('refdir',(1.,0.,0.));
#3104=DIRECTION('center_axis',(0.,0.,1.));
#3105=DIRECTION('ref_axis',(1.,0.,0.));
#3106=DIRECTION('center_axis',(0.,0.,-1.));
#3107=DIRECTION('ref_axis',(-1.,0.,0.));
#3108=DIRECTION('',(0.,0.,1.));
#3109=DIRECTION('center_axis',(0.,0.,-1.));
#3110=DIRECTION('ref_axis',(-1.,0.,0.));
#3111=DIRECTION('center_axis',(0.,-1.,0.));
#3112=DIRECTION('ref_axis',(0.,0.,-1.));
#3113=DIRECTION('',(0.,0.,1.));
#3114=DIRECTION('',(-1.,-1.22464679914735E-16,0.));
#3115=DIRECTION('',(0.,0.,1.));
#3116=DIRECTION('',(-1.,0.,0.));
#3117=DIRECTION('center_axis',(0.,-1.,0.));
#3118=DIRECTION('ref_axis',(0.,0.,-1.));
#3119=DIRECTION('',(0.,0.,1.));
#3120=DIRECTION('',(-1.,0.,0.));
#3121=DIRECTION('',(0.,0.,1.));
#3122=DIRECTION('',(-1.,-1.22464679914735E-16,0.));
#3123=DIRECTION('center_axis',(0.,-1.,0.));
#3124=DIRECTION('ref_axis',(0.,0.,-1.));
#3125=DIRECTION('',(0.,0.,1.));
#3126=DIRECTION('',(-1.,0.,0.));
#3127=DIRECTION('',(0.,0.,1.));
#3128=DIRECTION('',(-1.,-1.22464679914735E-16,0.));
#3129=DIRECTION('center_axis',(0.,-1.,0.));
#3130=DIRECTION('ref_axis',(0.,0.,-1.));
#3131=DIRECTION('',(0.,0.,1.));
#3132=DIRECTION('',(-1.,0.,0.));
#3133=DIRECTION('',(0.,0.,1.));
#3134=DIRECTION('',(-1.,-1.22464679914735E-16,0.));
#3135=DIRECTION('center_axis',(0.,-1.,0.));
#3136=DIRECTION('ref_axis',(0.,0.,-1.));
#3137=DIRECTION('',(0.,0.,1.));
#3138=DIRECTION('',(-1.,0.,0.));
#3139=DIRECTION('',(0.,0.,1.));
#3140=DIRECTION('',(-1.,-1.22464679914735E-16,0.));
#3141=DIRECTION('center_axis',(0.,-1.,0.));
#3142=DIRECTION('ref_axis',(0.,0.,-1.));
#3143=DIRECTION('',(0.,0.,1.));
#3144=DIRECTION('',(-1.,0.,0.));
#3145=DIRECTION('',(0.,0.,1.));
#3146=DIRECTION('',(-1.,-1.22464679914735E-16,0.));
#3147=DIRECTION('center_axis',(0.,-1.,0.));
#3148=DIRECTION('ref_axis',(0.,0.,-1.));
#3149=DIRECTION('',(0.,0.,1.));
#3150=DIRECTION('',(-1.,0.,0.));
#3151=DIRECTION('',(0.,0.,1.));
#3152=DIRECTION('',(-1.,-1.22464679914735E-16,0.));
#3153=DIRECTION('center_axis',(0.,-1.,0.));
#3154=DIRECTION('ref_axis',(0.,0.,-1.));
#3155=DIRECTION('',(0.,0.,1.));
#3156=DIRECTION('',(-1.,0.,0.));
#3157=DIRECTION('',(0.,0.,1.));
#3158=DIRECTION('',(-1.,-1.22464679914735E-16,0.));
#3159=DIRECTION('center_axis',(0.,-1.,0.));
#3160=DIRECTION('ref_axis',(0.,0.,-1.));
#3161=DIRECTION('',(0.,0.,1.));
#3162=DIRECTION('',(-1.,0.,0.));
#3163=DIRECTION('',(0.,0.,1.));
#3164=DIRECTION('',(-1.,-1.22464679914735E-16,0.));
#3165=DIRECTION('center_axis',(0.,-1.,0.));
#3166=DIRECTION('ref_axis',(0.,0.,-1.));
#3167=DIRECTION('',(-1.,0.,0.));
#3168=DIRECTION('',(0.,0.,1.));
#3169=DIRECTION('',(-1.,-1.22464679914735E-16,0.));
#3170=DIRECTION('',(0.,0.,-1.));
#3171=DIRECTION('center_axis',(0.,-1.,0.));
#3172=DIRECTION('ref_axis',(0.,0.,-1.));
#3173=DIRECTION('',(0.,0.,1.));
#3174=DIRECTION('',(-1.,0.,0.));
#3175=DIRECTION('',(0.,0.,-1.));
#3176=DIRECTION('',(-1.,-1.22464679914735E-16,0.));
#3177=DIRECTION('center_axis',(1.,0.,0.));
#3178=DIRECTION('ref_axis',(0.,0.,-1.));
#3179=DIRECTION('',(0.,-1.,0.));
#3180=DIRECTION('',(0.,0.,-1.));
#3181=DIRECTION('',(0.,-1.,0.));
#3182=DIRECTION('center_axis',(0.,-1.,0.));
#3183=DIRECTION('ref_axis',(0.,0.,-1.));
#3184=DIRECTION('',(-1.,0.,0.));
#3185=DIRECTION('',(0.,0.,1.));
#3186=DIRECTION('',(-1.,-1.22464679914735E-16,0.));
#3187=DIRECTION('center_axis',(0.,0.,-1.));
#3188=DIRECTION('ref_axis',(-1.,0.,0.));
#3189=DIRECTION('',(1.,0.,0.));
#3190=DIRECTION('',(1.,0.,0.));
#3191=DIRECTION('',(1.,0.,0.));
#3192=DIRECTION('',(1.,0.,0.));
#3193=DIRECTION('',(1.,0.,0.));
#3194=DIRECTION('',(1.,0.,0.));
#3195=DIRECTION('',(1.,0.,0.));
#3196=DIRECTION('',(1.,0.,0.));
#3197=DIRECTION('',(1.,0.,0.));
#3198=DIRECTION('',(1.,0.,0.));
#3199=DIRECTION('center_axis',(0.,0.,1.));
#3200=DIRECTION('ref_axis',(-1.,0.,0.));
#3201=DIRECTION('center_axis',(0.,0.,1.));
#3202=DIRECTION('ref_axis',(-1.,3.46944695195361E-15,0.));
#3203=DIRECTION('center_axis',(0.,0.,-1.));
#3204=DIRECTION('ref_axis',(-1.,0.,0.));
#3205=DIRECTION('',(-1.,0.,0.));
#3206=DIRECTION('',(-1.,0.,0.));
#3207=DIRECTION('',(-1.,0.,0.));
#3208=DIRECTION('',(-1.,0.,0.));
#3209=DIRECTION('',(-1.,0.,0.));
#3210=DIRECTION('',(-1.,0.,0.));
#3211=DIRECTION('',(-1.,0.,0.));
#3212=DIRECTION('',(-1.,0.,0.));
#3213=DIRECTION('',(-1.,0.,0.));
#3214=DIRECTION('',(-1.,0.,0.));
#3215=DIRECTION('center_axis',(0.,0.,-1.));
#3216=DIRECTION('ref_axis',(-1.,0.,0.));
#3217=DIRECTION('center_axis',(0.,0.,-1.));
#3218=DIRECTION('ref_axis',(-1.,0.,0.));
#3219=DIRECTION('center_axis',(0.,0.,1.));
#3220=DIRECTION('ref_axis',(1.,0.,0.));
#3221=DIRECTION('',(0.,0.,1.));
#3222=DIRECTION('center_axis',(0.,0.,1.));
#3223=DIRECTION('ref_axis',(-0.961769203083568,-0.273861278752579,0.));
#3224=DIRECTION('center_axis',(-1.,0.,0.));
#3225=DIRECTION('ref_axis',(0.,0.,1.));
#3226=DIRECTION('',(0.,-0.707106781186547,0.707106781186547));
#3227=DIRECTION('',(0.,0.707106781186548,0.707106781186548));
#3228=DIRECTION('center_axis',(0.,0.707106781186548,-0.707106781186548));
#3229=DIRECTION('ref_axis',(-1.,0.,0.));
#3230=DIRECTION('',(-0.577350269189626,-0.577350269189626,-0.577350269189626));
#3231=DIRECTION('center_axis',(-0.707106781186548,0.707106781186548,0.));
#3232=DIRECTION('ref_axis',(0.,0.,1.));
#3233=DIRECTION('',(-0.577350269189626,-0.577350269189626,0.577350269189626));
#3234=DIRECTION('center_axis',(0.,-0.707106781186548,-0.707106781186548));
#3235=DIRECTION('ref_axis',(1.,0.,0.));
#3236=DIRECTION('center_axis',(-1.,0.,0.));
#3237=DIRECTION('ref_axis',(0.,0.,1.));
#3238=DIRECTION('',(0.,-0.707106781186547,0.707106781186547));
#3239=DIRECTION('',(0.,0.707106781186548,0.707106781186548));
#3240=DIRECTION('center_axis',(0.,0.707106781186548,-0.707106781186548));
#3241=DIRECTION('ref_axis',(-1.,0.,0.));
#3242=DIRECTION('',(-0.577350269189626,-0.577350269189626,-0.577350269189626));
#3243=DIRECTION('center_axis',(-0.707106781186548,0.707106781186548,0.));
#3244=DIRECTION('ref_axis',(0.,0.,1.));
#3245=DIRECTION('',(-0.577350269189626,-0.577350269189626,0.577350269189626));
#3246=DIRECTION('center_axis',(0.,-0.707106781186548,-0.707106781186548));
#3247=DIRECTION('ref_axis',(1.,0.,0.));
#3248=DIRECTION('center_axis',(-1.,0.,0.));
#3249=DIRECTION('ref_axis',(0.,0.,1.));
#3250=DIRECTION('',(0.,-0.707106781186547,0.707106781186547));
#3251=DIRECTION('',(0.,0.707106781186548,0.707106781186548));
#3252=DIRECTION('center_axis',(0.,0.707106781186548,-0.707106781186548));
#3253=DIRECTION('ref_axis',(-1.,0.,0.));
#3254=DIRECTION('',(-0.577350269189626,-0.577350269189626,-0.577350269189626));
#3255=DIRECTION('center_axis',(-0.707106781186548,0.707106781186548,0.));
#3256=DIRECTION('ref_axis',(0.,0.,1.));
#3257=DIRECTION('',(-0.577350269189626,-0.577350269189626,0.577350269189626));
#3258=DIRECTION('center_axis',(0.,-0.707106781186548,-0.707106781186548));
#3259=DIRECTION('ref_axis',(1.,0.,0.));
#3260=DIRECTION('center_axis',(-1.,0.,0.));
#3261=DIRECTION('ref_axis',(0.,0.,1.));
#3262=DIRECTION('',(0.,-0.707106781186547,0.707106781186547));
#3263=DIRECTION('',(0.,0.707106781186548,0.707106781186548));
#3264=DIRECTION('center_axis',(0.,0.707106781186548,-0.707106781186548));
#3265=DIRECTION('ref_axis',(-1.,0.,0.));
#3266=DIRECTION('',(-0.577350269189626,-0.577350269189626,-0.577350269189626));
#3267=DIRECTION('center_axis',(-0.707106781186548,0.707106781186548,0.));
#3268=DIRECTION('ref_axis',(0.,0.,1.));
#3269=DIRECTION('',(-0.577350269189626,-0.577350269189626,0.577350269189626));
#3270=DIRECTION('center_axis',(0.,-0.707106781186548,-0.707106781186548));
#3271=DIRECTION('ref_axis',(1.,0.,0.));
#3272=DIRECTION('center_axis',(-1.,0.,0.));
#3273=DIRECTION('ref_axis',(0.,0.,1.));
#3274=DIRECTION('',(0.,-0.707106781186547,0.707106781186547));
#3275=DIRECTION('',(0.,0.707106781186548,0.707106781186548));
#3276=DIRECTION('center_axis',(0.,0.707106781186548,-0.707106781186548));
#3277=DIRECTION('ref_axis',(-1.,0.,0.));
#3278=DIRECTION('',(-0.577350269189626,-0.577350269189626,-0.577350269189626));
#3279=DIRECTION('center_axis',(-0.707106781186548,0.707106781186548,0.));
#3280=DIRECTION('ref_axis',(0.,0.,1.));
#3281=DIRECTION('',(-0.577350269189626,-0.577350269189626,0.577350269189626));
#3282=DIRECTION('center_axis',(0.,-0.707106781186548,-0.707106781186548));
#3283=DIRECTION('ref_axis',(1.,0.,0.));
#3284=DIRECTION('center_axis',(-1.,0.,0.));
#3285=DIRECTION('ref_axis',(0.,0.,1.));
#3286=DIRECTION('',(0.,-0.707106781186547,0.707106781186547));
#3287=DIRECTION('',(0.,0.707106781186548,0.707106781186548));
#3288=DIRECTION('center_axis',(0.,0.707106781186548,-0.707106781186548));
#3289=DIRECTION('ref_axis',(-1.,0.,0.));
#3290=DIRECTION('',(-0.577350269189626,-0.577350269189626,-0.577350269189626));
#3291=DIRECTION('center_axis',(-0.707106781186548,0.707106781186548,0.));
#3292=DIRECTION('ref_axis',(0.,0.,1.));
#3293=DIRECTION('',(-0.577350269189626,-0.577350269189626,0.577350269189626));
#3294=DIRECTION('center_axis',(0.,-0.707106781186548,-0.707106781186548));
#3295=DIRECTION('ref_axis',(1.,0.,0.));
#3296=DIRECTION('center_axis',(-1.,0.,0.));
#3297=DIRECTION('ref_axis',(0.,0.,1.));
#3298=DIRECTION('',(0.,-0.707106781186547,0.707106781186547));
#3299=DIRECTION('',(0.,0.707106781186548,0.707106781186548));
#3300=DIRECTION('center_axis',(0.,0.707106781186548,-0.707106781186548));
#3301=DIRECTION('ref_axis',(-1.,0.,0.));
#3302=DIRECTION('',(-0.577350269189626,-0.577350269189626,-0.577350269189626));
#3303=DIRECTION('center_axis',(-0.707106781186548,0.707106781186548,0.));
#3304=DIRECTION('ref_axis',(0.,0.,1.));
#3305=DIRECTION('',(-0.577350269189626,-0.577350269189626,0.577350269189626));
#3306=DIRECTION('center_axis',(0.,-0.707106781186548,-0.707106781186548));
#3307=DIRECTION('ref_axis',(1.,0.,0.));
#3308=DIRECTION('center_axis',(-1.,0.,0.));
#3309=DIRECTION('ref_axis',(0.,0.,1.));
#3310=DIRECTION('',(0.,-0.707106781186547,0.707106781186547));
#3311=DIRECTION('',(0.,0.707106781186548,0.707106781186548));
#3312=DIRECTION('center_axis',(0.,0.707106781186548,-0.707106781186548));
#3313=DIRECTION('ref_axis',(-1.,0.,0.));
#3314=DIRECTION('',(-0.577350269189626,-0.577350269189626,-0.577350269189626));
#3315=DIRECTION('center_axis',(-0.707106781186548,0.707106781186548,0.));
#3316=DIRECTION('ref_axis',(0.,0.,1.));
#3317=DIRECTION('',(-0.577350269189626,-0.577350269189626,0.577350269189626));
#3318=DIRECTION('center_axis',(0.,-0.707106781186548,-0.707106781186548));
#3319=DIRECTION('ref_axis',(1.,0.,0.));
#3320=DIRECTION('center_axis',(-1.,0.,0.));
#3321=DIRECTION('ref_axis',(0.,0.,1.));
#3322=DIRECTION('',(0.,-0.707106781186547,0.707106781186547));
#3323=DIRECTION('',(0.,0.707106781186548,0.707106781186548));
#3324=DIRECTION('center_axis',(0.,0.707106781186548,-0.707106781186548));
#3325=DIRECTION('ref_axis',(-1.,0.,0.));
#3326=DIRECTION('',(-0.577350269189626,-0.577350269189626,-0.577350269189626));
#3327=DIRECTION('center_axis',(-0.707106781186548,0.707106781186548,0.));
#3328=DIRECTION('ref_axis',(0.,0.,1.));
#3329=DIRECTION('',(-0.577350269189626,-0.577350269189626,0.577350269189626));
#3330=DIRECTION('center_axis',(0.,-0.707106781186548,-0.707106781186548));
#3331=DIRECTION('ref_axis',(1.,0.,0.));
#3332=DIRECTION('center_axis',(-1.,0.,0.));
#3333=DIRECTION('ref_axis',(0.,0.,1.));
#3334=DIRECTION('',(0.,-0.707106781186547,0.707106781186547));
#3335=DIRECTION('',(0.,0.707106781186548,0.707106781186548));
#3336=DIRECTION('center_axis',(0.,0.707106781186548,-0.707106781186548));
#3337=DIRECTION('ref_axis',(-1.,0.,0.));
#3338=DIRECTION('',(-0.577350269189626,-0.577350269189626,-0.577350269189626));
#3339=DIRECTION('center_axis',(-0.707106781186548,0.707106781186548,0.));
#3340=DIRECTION('ref_axis',(0.,0.,1.));
#3341=DIRECTION('',(-0.577350269189626,-0.577350269189626,0.577350269189626));
#3342=DIRECTION('center_axis',(0.,-0.707106781186548,-0.707106781186548));
#3343=DIRECTION('ref_axis',(1.,0.,0.));
#9283=CARTESIAN_POINT('',(0.,0.,0.));
#9284=CARTESIAN_POINT('Origin',(0.,0.,-4.5));
#9285=CARTESIAN_POINT('',(-1.25,-1.53080849893419E-16,-0.5));
#9286=CARTESIAN_POINT('Origin',(0.,0.,-0.5));
#9287=CARTESIAN_POINT('',(-1.25,-1.53080849893419E-16,0.5));
#9288=CARTESIAN_POINT('',(-1.25,-1.53080849893419E-16,-4.5));
#9289=CARTESIAN_POINT('Origin',(0.,0.,0.5));
#9290=CARTESIAN_POINT('Origin',(0.,-2.,0.5));
#9291=CARTESIAN_POINT('',(-17.1201286922563,-2.,-0.5));
#9292=CARTESIAN_POINT('',(-17.1201286922563,-2.,0.5));
#9293=CARTESIAN_POINT('',(-17.1201286922563,-2.,-0.5));
#9294=CARTESIAN_POINT('',(-17.6201286922563,-2.,0.5));
#9295=CARTESIAN_POINT('',(2.44929359829471E-16,-2.,0.5));
#9296=CARTESIAN_POINT('',(-17.6201286922563,-2.,-0.5));
#9297=CARTESIAN_POINT('',(-17.6201286922563,-2.,-0.5));
#9298=CARTESIAN_POINT('',(0.,-2.,-0.5));
#9299=CARTESIAN_POINT('Origin',(0.,-2.,0.5));
#9300=CARTESIAN_POINT('',(-16.6201286922563,-2.,-0.5));
#9301=CARTESIAN_POINT('',(-16.6201286922563,-2.,0.5));
#9302=CARTESIAN_POINT('',(-16.6201286922563,-2.,-0.5));
#9303=CARTESIAN_POINT('',(-16.1201286922563,-2.,-0.5));
#9304=CARTESIAN_POINT('',(0.,-2.,-0.5));
#9305=CARTESIAN_POINT('',(-16.1201286922563,-2.,0.5));
#9306=CARTESIAN_POINT('',(-16.1201286922563,-2.,-0.5));
#9307=CARTESIAN_POINT('',(2.44929359829471E-16,-2.,0.5));
#9308=CARTESIAN_POINT('Origin',(0.,-2.,0.5));
#9309=CARTESIAN_POINT('',(-15.6201286922563,-2.,-0.5));
#9310=CARTESIAN_POINT('',(-15.6201286922563,-2.,0.5));
#9311=CARTESIAN_POINT('',(-15.6201286922563,-2.,-0.5));
#9312=CARTESIAN_POINT('',(-15.1201286922563,-2.,-0.5));
#9313=CARTESIAN_POINT('',(0.,-2.,-0.5));
#9314=CARTESIAN_POINT('',(-15.1201286922563,-2.,0.5));
#9315=CARTESIAN_POINT('',(-15.1201286922563,-2.,-0.5));
#9316=CARTESIAN_POINT('',(2.44929359829471E-16,-2.,0.5));
#9317=CARTESIAN_POINT('Origin',(0.,-2.,0.5));
#9318=CARTESIAN_POINT('',(-14.6201286922563,-2.,-0.5));
#9319=CARTESIAN_POINT('',(-14.6201286922563,-2.,0.5));
#9320=CARTESIAN_POINT('',(-14.6201286922563,-2.,-0.5));
#9321=CARTESIAN_POINT('',(-14.1201286922563,-2.,-0.5));
#9322=CARTESIAN_POINT('',(0.,-2.,-0.5));
#9323=CARTESIAN_POINT('',(-14.1201286922563,-2.,0.5));
#9324=CARTESIAN_POINT('',(-14.1201286922563,-2.,-0.5));
#9325=CARTESIAN_POINT('',(2.44929359829471E-16,-2.,0.5));
#9326=CARTESIAN_POINT('Origin',(0.,-2.,0.5));
#9327=CARTESIAN_POINT('',(-13.6201286922563,-2.,-0.5));
#9328=CARTESIAN_POINT('',(-13.6201286922563,-2.,0.5));
#9329=CARTESIAN_POINT('',(-13.6201286922563,-2.,-0.5));
#9330=CARTESIAN_POINT('',(-13.1201286922563,-2.,-0.5));
#9331=CARTESIAN_POINT('',(0.,-2.,-0.5));
#9332=CARTESIAN_POINT('',(-13.1201286922563,-2.,0.5));
#9333=CARTESIAN_POINT('',(-13.1201286922563,-2.,-0.5));
#9334=CARTESIAN_POINT('',(2.44929359829471E-16,-2.,0.5));
#9335=CARTESIAN_POINT('Origin',(0.,-2.,0.5));
#9336=CARTESIAN_POINT('',(-12.6201286922563,-2.,-0.5));
#9337=CARTESIAN_POINT('',(-12.6201286922563,-2.,0.5));
#9338=CARTESIAN_POINT('',(-12.6201286922563,-2.,-0.5));
#9339=CARTESIAN_POINT('',(-12.1201286922563,-2.,-0.5));
#9340=CARTESIAN_POINT('',(0.,-2.,-0.5));
#9341=CARTESIAN_POINT('',(-12.1201286922563,-2.,0.5));
#9342=CARTESIAN_POINT('',(-12.1201286922563,-2.,-0.5));
#9343=CARTESIAN_POINT('',(2.44929359829471E-16,-2.,0.5));
#9344=CARTESIAN_POINT('Origin',(0.,-2.,0.5));
#9345=CARTESIAN_POINT('',(-11.6201286922563,-2.,-0.5));
#9346=CARTESIAN_POINT('',(-11.6201286922563,-2.,0.5));
#9347=CARTESIAN_POINT('',(-11.6201286922563,-2.,-0.5));
#9348=CARTESIAN_POINT('',(-11.1201286922563,-2.,-0.5));
#9349=CARTESIAN_POINT('',(0.,-2.,-0.5));
#9350=CARTESIAN_POINT('',(-11.1201286922563,-2.,0.5));
#9351=CARTESIAN_POINT('',(-11.1201286922563,-2.,-0.5));
#9352=CARTESIAN_POINT('',(2.44929359829471E-16,-2.,0.5));
#9353=CARTESIAN_POINT('Origin',(0.,-2.,0.5));
#9354=CARTESIAN_POINT('',(-10.6201286922563,-2.,-0.5));
#9355=CARTESIAN_POINT('',(-10.6201286922563,-2.,0.5));
#9356=CARTESIAN_POINT('',(-10.6201286922563,-2.,-0.5));
#9357=CARTESIAN_POINT('',(-10.1201286922563,-2.,-0.5));
#9358=CARTESIAN_POINT('',(0.,-2.,-0.5));
#9359=CARTESIAN_POINT('',(-10.1201286922563,-2.,0.5));
#9360=CARTESIAN_POINT('',(-10.1201286922563,-2.,-0.5));
#9361=CARTESIAN_POINT('',(2.44929359829471E-16,-2.,0.5));
#9362=CARTESIAN_POINT('Origin',(0.,-2.,0.5));
#9363=CARTESIAN_POINT('',(-9.6201286922563,-2.,-0.5));
#9364=CARTESIAN_POINT('',(-9.6201286922563,-2.,0.5));
#9365=CARTESIAN_POINT('',(-9.6201286922563,-2.,-0.5));
#9366=CARTESIAN_POINT('',(-9.1201286922563,-2.,-0.5));
#9367=CARTESIAN_POINT('',(0.,-2.,-0.5));
#9368=CARTESIAN_POINT('',(-9.1201286922563,-2.,0.5));
#9369=CARTESIAN_POINT('',(-9.1201286922563,-2.,-0.5));
#9370=CARTESIAN_POINT('',(2.44929359829471E-16,-2.,0.5));
#9371=CARTESIAN_POINT('Origin',(0.,-2.,0.5));
#9372=CARTESIAN_POINT('',(-18.1201286922563,-2.,-0.5));
#9373=CARTESIAN_POINT('',(-18.3701286922563,-2.,-0.5));
#9374=CARTESIAN_POINT('',(0.,-2.,-0.5));
#9375=CARTESIAN_POINT('',(-18.1201286922563,-2.,0.5));
#9376=CARTESIAN_POINT('',(-18.1201286922563,-2.,-0.5));
#9377=CARTESIAN_POINT('',(-18.3701286922563,-2.,0.5));
#9378=CARTESIAN_POINT('',(2.44929359829471E-16,-2.,0.5));
#9379=CARTESIAN_POINT('',(-18.3701286922563,-2.,0.5));
#9380=CARTESIAN_POINT('Origin',(0.,-2.,0.5));
#9381=CARTESIAN_POINT('',(-8.6201286922563,-2.,-0.5));
#9382=CARTESIAN_POINT('',(-8.6201286922563,-2.,0.5));
#9383=CARTESIAN_POINT('',(-8.6201286922563,-2.,-0.5));
#9384=CARTESIAN_POINT('',(3.,-2.,-0.5));
#9385=CARTESIAN_POINT('',(0.,-2.,-0.5));
#9386=CARTESIAN_POINT('',(3.,-2.,0.5));
#9387=CARTESIAN_POINT('',(3.,-2.,0.5));
#9388=CARTESIAN_POINT('',(2.44929359829471E-16,-2.,0.5));
#9389=CARTESIAN_POINT('Origin',(3.,2.,0.5));
#9390=CARTESIAN_POINT('',(3.,2.,-0.5));
#9391=CARTESIAN_POINT('',(3.,2.,-0.5));
#9392=CARTESIAN_POINT('',(3.,2.,0.5));
#9393=CARTESIAN_POINT('',(3.,2.,0.5));
#9394=CARTESIAN_POINT('',(3.,2.,0.5));
#9395=CARTESIAN_POINT('Origin',(0.,2.,0.5));
#9396=CARTESIAN_POINT('',(-7.83447493940356,2.,-0.5));
#9397=CARTESIAN_POINT('',(0.,2.,-0.5));
#9398=CARTESIAN_POINT('',(-7.83447493940357,2.,0.5));
#9399=CARTESIAN_POINT('',(-7.83447493940356,2.,0.5));
#9400=CARTESIAN_POINT('',(-2.44929359829471E-16,2.,0.5));
#9401=CARTESIAN_POINT('Origin',(0.,0.,0.5));
#9402=CARTESIAN_POINT('',(0.,-2.,0.5));
#9403=CARTESIAN_POINT('',(1.,-2.,0.5));
#9404=CARTESIAN_POINT('',(2.,-2.,0.5));
#9405=CARTESIAN_POINT('',(3.,-2.,0.5));
#9406=CARTESIAN_POINT('',(4.,-2.,0.5));
#9407=CARTESIAN_POINT('',(5.,-2.,0.5));
#9408=CARTESIAN_POINT('',(6.,-2.,0.5));
#9409=CARTESIAN_POINT('',(7.,-2.,0.5));
#9410=CARTESIAN_POINT('',(8.,-2.,0.5));
#9411=CARTESIAN_POINT('',(9.,-2.,0.5));
#9412=CARTESIAN_POINT('',(-18.6335200360776,-1.075,0.5));
#9413=CARTESIAN_POINT('Origin',(-7.83447493940356,-18.5,0.5));
#9414=CARTESIAN_POINT('Origin',(-18.3701286922563,-1.5,0.5));
#9415=CARTESIAN_POINT('Origin',(0.,0.,-0.5));
#9416=CARTESIAN_POINT('',(-9.1201286922563,-2.,-0.5));
#9417=CARTESIAN_POINT('',(-10.1201286922563,-2.,-0.5));
#9418=CARTESIAN_POINT('',(-11.1201286922563,-2.,-0.5));
#9419=CARTESIAN_POINT('',(-12.1201286922563,-2.,-0.5));
#9420=CARTESIAN_POINT('',(-13.1201286922563,-2.,-0.5));
#9421=CARTESIAN_POINT('',(-14.1201286922563,-2.,-0.5));
#9422=CARTESIAN_POINT('',(-15.1201286922563,-2.,-0.5));
#9423=CARTESIAN_POINT('',(-16.1201286922563,-2.,-0.5));
#9424=CARTESIAN_POINT('',(-17.1201286922563,-2.,-0.5));
#9425=CARTESIAN_POINT('',(-18.1201286922563,-2.,-0.5));
#9426=CARTESIAN_POINT('',(-18.6335200360776,-1.075,-0.5));
#9427=CARTESIAN_POINT('Origin',(-18.3701286922563,-1.5,-0.5));
#9428=CARTESIAN_POINT('Origin',(-7.83447493940356,-18.5,-0.5));
#9429=CARTESIAN_POINT('Origin',(-7.83447493940356,-18.5,0.5));
#9430=CARTESIAN_POINT('',(-18.6335200360776,-1.075,0.5));
#9431=CARTESIAN_POINT('Origin',(-18.3701286922563,-1.5,0.5));
#9432=CARTESIAN_POINT('Origin',(-18.1201286922563,-2.,-0.5));
#9433=CARTESIAN_POINT('',(-18.1201286922563,-2.5,-4.33680868994202E-16));
#9434=CARTESIAN_POINT('',(-18.1201286922563,-2.,-0.5));
#9435=CARTESIAN_POINT('',(-18.1201286922563,-2.5,-2.16840434497101E-16));
#9436=CARTESIAN_POINT('Origin',(-17.6201286922563,-2.5,-4.33680868994202E-16));
#9437=CARTESIAN_POINT('',(-17.9534620255896,-2.33333333333333,0.166666666666666));
#9438=CARTESIAN_POINT('Origin',(-18.1201286922563,-2.5,-0.5));
#9439=CARTESIAN_POINT('',(-17.9534620255896,-2.33333333333333,-0.166666666666666));
#9440=CARTESIAN_POINT('Origin',(0.,-2.,-0.5));
#9441=CARTESIAN_POINT('Origin',(-9.1201286922563,-2.,-0.5));
#9442=CARTESIAN_POINT('',(-9.1201286922563,-2.5,-4.33680868994202E-16));
#9443=CARTESIAN_POINT('',(-9.1201286922563,-2.,-0.5));
#9444=CARTESIAN_POINT('',(-9.1201286922563,-2.5,-2.16840434497101E-16));
#9445=CARTESIAN_POINT('Origin',(-8.6201286922563,-2.5,-4.33680868994202E-16));
#9446=CARTESIAN_POINT('',(-8.95346202558963,-2.33333333333333,0.166666666666666));
#9447=CARTESIAN_POINT('Origin',(-9.1201286922563,-2.5,-0.5));
#9448=CARTESIAN_POINT('',(-8.95346202558963,-2.33333333333333,-0.166666666666666));
#9449=CARTESIAN_POINT('Origin',(9.,-2.,-0.5));
#9450=CARTESIAN_POINT('Origin',(-10.1201286922563,-2.,-0.5));
#9451=CARTESIAN_POINT('',(-10.1201286922563,-2.5,-4.33680868994202E-16));
#9452=CARTESIAN_POINT('',(-10.1201286922563,-2.,-0.5));
#9453=CARTESIAN_POINT('',(-10.1201286922563,-2.5,-2.16840434497101E-16));
#9454=CARTESIAN_POINT('Origin',(-9.6201286922563,-2.5,-4.33680868994202E-16));
#9455=CARTESIAN_POINT('',(-9.95346202558963,-2.33333333333333,0.166666666666666));
#9456=CARTESIAN_POINT('Origin',(-10.1201286922563,-2.5,-0.5));
#9457=CARTESIAN_POINT('',(-9.95346202558963,-2.33333333333333,-0.166666666666666));
#9458=CARTESIAN_POINT('Origin',(8.,-2.,-0.5));
#9459=CARTESIAN_POINT('Origin',(-11.1201286922563,-2.,-0.5));
#9460=CARTESIAN_POINT('',(-11.1201286922563,-2.5,-4.33680868994202E-16));
#9461=CARTESIAN_POINT('',(-11.1201286922563,-2.,-0.5));
#9462=CARTESIAN_POINT('',(-11.1201286922563,-2.5,-2.16840434497101E-16));
#9463=CARTESIAN_POINT('Origin',(-10.6201286922563,-2.5,-4.33680868994202E-16));
#9464=CARTESIAN_POINT('',(-10.9534620255896,-2.33333333333333,0.166666666666666));
#9465=CARTESIAN_POINT('Origin',(-11.1201286922563,-2.5,-0.5));
#9466=CARTESIAN_POINT('',(-10.9534620255896,-2.33333333333333,-0.166666666666666));
#9467=CARTESIAN_POINT('Origin',(7.,-2.,-0.5));
#9468=CARTESIAN_POINT('Origin',(-12.1201286922563,-2.,-0.5));
#9469=CARTESIAN_POINT('',(-12.1201286922563,-2.5,-4.33680868994202E-16));
#9470=CARTESIAN_POINT('',(-12.1201286922563,-2.,-0.5));
#9471=CARTESIAN_POINT('',(-12.1201286922563,-2.5,-2.16840434497101E-16));
#9472=CARTESIAN_POINT('Origin',(-11.6201286922563,-2.5,-4.33680868994202E-16));
#9473=CARTESIAN_POINT('',(-11.9534620255896,-2.33333333333333,0.166666666666666));
#9474=CARTESIAN_POINT('Origin',(-12.1201286922563,-2.5,-0.5));
#9475=CARTESIAN_POINT('',(-11.9534620255896,-2.33333333333333,-0.166666666666666));
#9476=CARTESIAN_POINT('Origin',(6.,-2.,-0.5));
#9477=CARTESIAN_POINT('Origin',(-13.1201286922563,-2.,-0.5));
#9478=CARTESIAN_POINT('',(-13.1201286922563,-2.5,-4.33680868994202E-16));
#9479=CARTESIAN_POINT('',(-13.1201286922563,-2.,-0.5));
#9480=CARTESIAN_POINT('',(-13.1201286922563,-2.5,-2.16840434497101E-16));
#9481=CARTESIAN_POINT('Origin',(-12.6201286922563,-2.5,-4.33680868994202E-16));
#9482=CARTESIAN_POINT('',(-12.9534620255896,-2.33333333333333,0.166666666666666));
#9483=CARTESIAN_POINT('Origin',(-13.1201286922563,-2.5,-0.5));
#9484=CARTESIAN_POINT('',(-12.9534620255896,-2.33333333333333,-0.166666666666666));
#9485=CARTESIAN_POINT('Origin',(5.,-2.,-0.5));
#9486=CARTESIAN_POINT('Origin',(-14.1201286922563,-2.,-0.5));
#9487=CARTESIAN_POINT('',(-14.1201286922563,-2.5,-4.33680868994202E-16));
#9488=CARTESIAN_POINT('',(-14.1201286922563,-2.,-0.5));
#9489=CARTESIAN_POINT('',(-14.1201286922563,-2.5,-2.16840434497101E-16));
#9490=CARTESIAN_POINT('Origin',(-13.6201286922563,-2.5,-4.33680868994202E-16));
#9491=CARTESIAN_POINT('',(-13.9534620255896,-2.33333333333333,0.166666666666666));
#9492=CARTESIAN_POINT('Origin',(-14.1201286922563,-2.5,-0.5));
#9493=CARTESIAN_POINT('',(-13.9534620255896,-2.33333333333333,-0.166666666666666));
#9494=CARTESIAN_POINT('Origin',(4.,-2.,-0.5));
#9495=CARTESIAN_POINT('Origin',(-15.1201286922563,-2.,-0.5));
#9496=CARTESIAN_POINT('',(-15.1201286922563,-2.5,-4.33680868994202E-16));
#9497=CARTESIAN_POINT('',(-15.1201286922563,-2.,-0.5));
#9498=CARTESIAN_POINT('',(-15.1201286922563,-2.5,-2.16840434497101E-16));
#9499=CARTESIAN_POINT('Origin',(-14.6201286922563,-2.5,-4.33680868994202E-16));
#9500=CARTESIAN_POINT('',(-14.9534620255896,-2.33333333333333,0.166666666666666));
#9501=CARTESIAN_POINT('Origin',(-15.1201286922563,-2.5,-0.5));
#9502=CARTESIAN_POINT('',(-14.9534620255896,-2.33333333333333,-0.166666666666666));
#9503=CARTESIAN_POINT('Origin',(3.,-2.,-0.5));
#9504=CARTESIAN_POINT('Origin',(-16.1201286922563,-2.,-0.5));
#9505=CARTESIAN_POINT('',(-16.1201286922563,-2.5,-4.33680868994202E-16));
#9506=CARTESIAN_POINT('',(-16.1201286922563,-2.,-0.5));
#9507=CARTESIAN_POINT('',(-16.1201286922563,-2.5,-2.16840434497101E-16));
#9508=CARTESIAN_POINT('Origin',(-15.6201286922563,-2.5,-4.33680868994202E-16));
#9509=CARTESIAN_POINT('',(-15.9534620255896,-2.33333333333333,0.166666666666666));
#9510=CARTESIAN_POINT('Origin',(-16.1201286922563,-2.5,-0.5));
#9511=CARTESIAN_POINT('',(-15.9534620255896,-2.33333333333333,-0.166666666666666));
#9512=CARTESIAN_POINT('Origin',(2.,-2.,-0.5));
#9513=CARTESIAN_POINT('Origin',(-17.1201286922563,-2.,-0.5));
#9514=CARTESIAN_POINT('',(-17.1201286922563,-2.5,-4.33680868994202E-16));
#9515=CARTESIAN_POINT('',(-17.1201286922563,-2.,-0.5));
#9516=CARTESIAN_POINT('',(-17.1201286922563,-2.5,-2.16840434497101E-16));
#9517=CARTESIAN_POINT('Origin',(-16.6201286922563,-2.5,-4.33680868994202E-16));
#9518=CARTESIAN_POINT('',(-16.9534620255896,-2.33333333333333,0.166666666666666));
#9519=CARTESIAN_POINT('Origin',(-17.1201286922563,-2.5,-0.5));
#9520=CARTESIAN_POINT('',(-16.9534620255896,-2.33333333333333,-0.166666666666666));
#9521=CARTESIAN_POINT('Origin',(1.,-2.,-0.5));
#9550=UNCERTAINTY_MEASURE_WITH_UNIT(LENGTH_MEASURE(0.01),#9562,
'DISTANCE_ACCURACY_VALUE',
'Maximum model space distance between geometric entities at asserted c
onnectivities');
#9553=UNCERTAINTY_MEASURE_WITH_UNIT(LENGTH_MEASURE(0.01),#9562,
'DISTANCE_ACCURACY_VALUE',
'Maximum model space distance between geometric entities at asserted c
onnectivities');
#9558=(
GEOMETRIC_REPRESENTATION_CONTEXT(3)
GLOBAL_UNCERTAINTY_ASSIGNED_CONTEXT((#9550))
GLOBAL_UNIT_ASSIGNED_CONTEXT((#9562,#9564,#9565))
REPRESENTATION_CONTEXT('','3D')
);
#9561=(
GEOMETRIC_REPRESENTATION_CONTEXT(3)
GLOBAL_UNCERTAINTY_ASSIGNED_CONTEXT((#9553))
GLOBAL_UNIT_ASSIGNED_CONTEXT((#9562,#9564,#9565))
REPRESENTATION_CONTEXT('','3D')
);
#9562=(
LENGTH_UNIT()
NAMED_UNIT(*)
SI_UNIT(.MILLI.,.METRE.)
);
#9564=(
NAMED_UNIT(*)
PLANE_ANGLE_UNIT()
SI_UNIT($,.RADIAN.)
);
#9565=(
NAMED_UNIT(*)
SI_UNIT($,.STERADIAN.)
SOLID_ANGLE_UNIT()
);
#9570=SHAPE_DEFINITION_REPRESENTATION(#9577,#9590);
#9577=PRODUCT_DEFINITION_SHAPE('',$,#9598);
#9590=SHAPE_REPRESENTATION('',(#2613),#9558);
#9593=PRODUCT_DEFINITION_CONTEXT('part definition',#9616,'design');
#9598=PRODUCT_DEFINITION('foil cutter','foil cutter',#9605,#9593);
#9605=PRODUCT_DEFINITION_FORMATION('',$,#9622);
#9616=APPLICATION_CONTEXT(
'Core Data for Automotive Mechanical Design Process');
#9617=PRODUCT_CONTEXT('part definition',#9616,'mechanical');
#9622=PRODUCT('foil cutter','foil cutter',$,(#9617));
#9626=PRESENTATION_STYLE_ASSIGNMENT((#9631));
#9631=SURFACE_STYLE_USAGE(.BOTH.,#9636);
#9636=SURFACE_SIDE_STYLE('',(#9641));
#9641=SURFACE_STYLE_FILL_AREA(#9646);
#9646=FILL_AREA_STYLE('Opaque(61,176,222)',(#9651));
#9651=FILL_AREA_STYLE_COLOUR('Opaque(61,176,222)',#9656);
#9656=COLOUR_RGB('Opaque(61,176,222)',0.23921568627451,0.690196078431373,
0.870588235294118);
ENDSEC;
END-ISO-10303-21;
